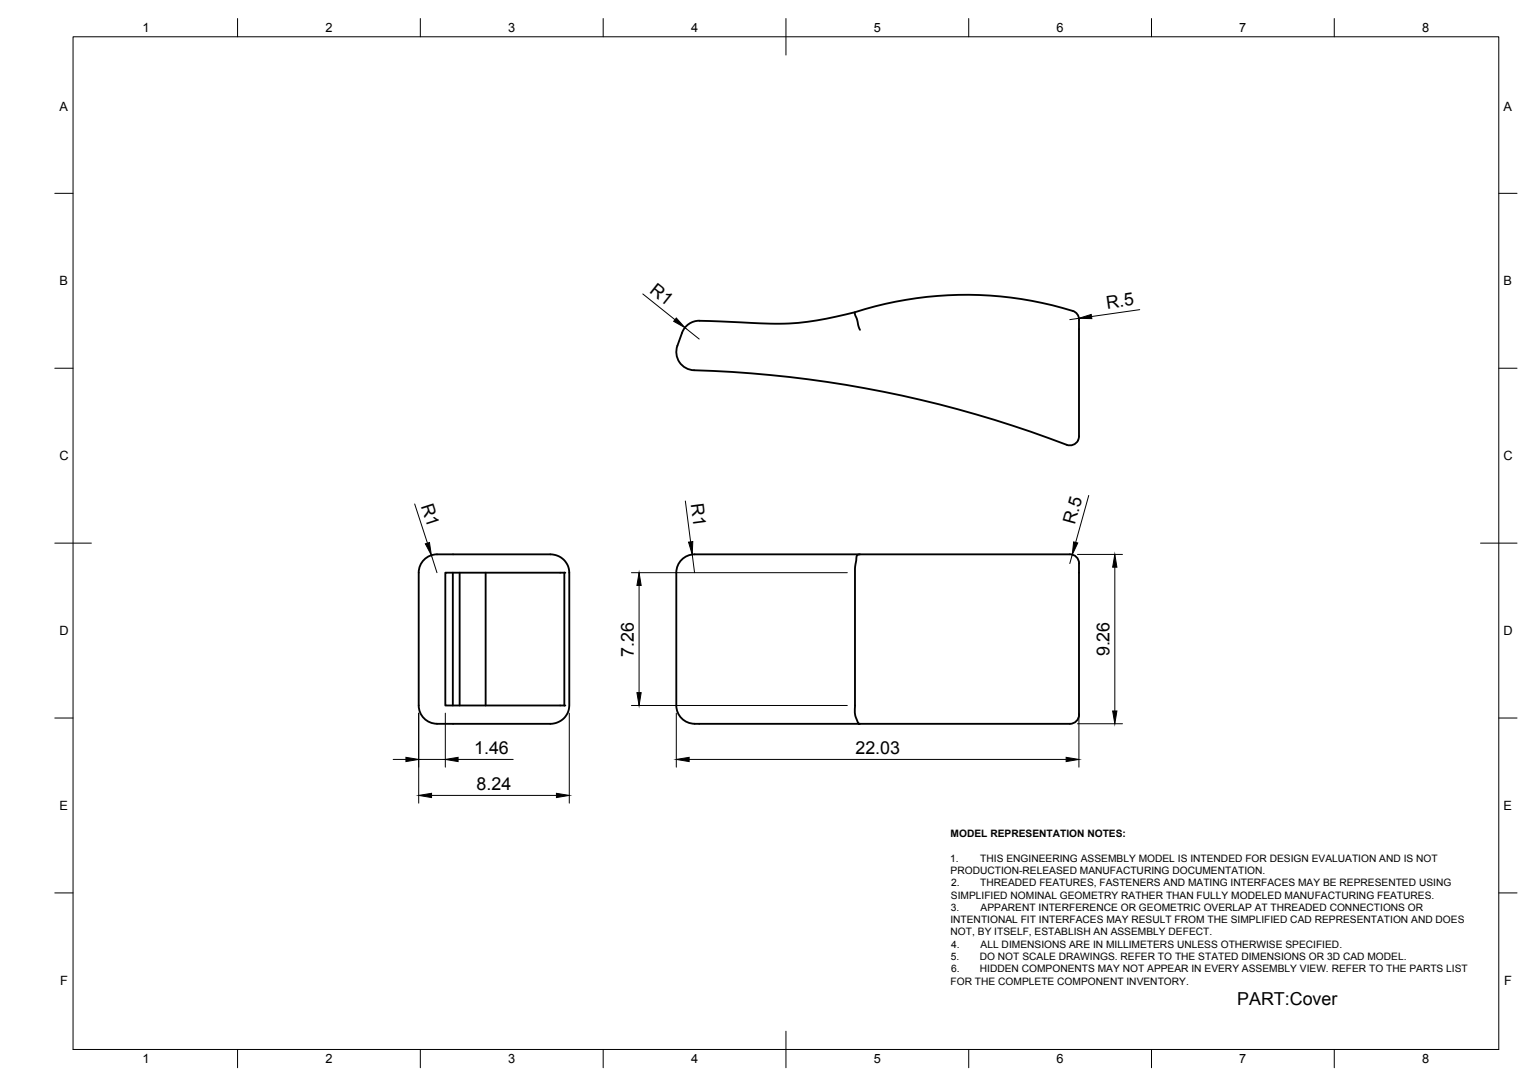
ISO-10303-21;
HEADER;
/* Generated by software containing ST-Developer
 * from STEP Tools, Inc. (www.steptools.com) 
 */

FILE_DESCRIPTION(
/* description */ (''),
/* implementation_level */ '2;1');

FILE_NAME(
/* name */ 'Cover.step',
/* time_stamp */ '2026-10-05T16:20:14-07:00',
/* author */ (''),
/* organization */ (''),
/* preprocessor_version */ 'ST-DEVELOPER v20.2',
/* originating_system */ 'Autodesk Translation Framework v15.15.0.0',
/* authorisation */ '');

FILE_SCHEMA (('AUTOMOTIVE_DESIGN { 1 0 10303 214 3 1 1 }'));
ENDSEC;

DATA;
#10=MECHANICAL_DESIGN_GEOMETRIC_PRESENTATION_REPRESENTATION('',(#255),#23577);
#47=SPHERICAL_SURFACE('',#4635,1.);
#48=SPHERICAL_SURFACE('',#4644,1.);
#49=SPHERICAL_SURFACE('',#4650,1.);
#50=SPHERICAL_SURFACE('',#4654,1.);
#62=B_SPLINE_SURFACE_WITH_KNOTS('',3,3,((#22693,#22694,#22695,#22696,#22697,
#22698),(#22699,#22700,#22701,#22702,#22703,#22704),(#22705,#22706,#22707,
#22708,#22709,#22710),(#22711,#22712,#22713,#22714,#22715,#22716),(#22717,
#22718,#22719,#22720,#22721,#22722),(#22723,#22724,#22725,#22726,#22727,
#22728)),.UNSPECIFIED.,.F.,.F.,.F.,(4,1,1,4),(4,1,1,4),(0.,0.285714285714286,
0.571428571428571,1.00003411570466),(-3.41157046611592E-5,0.0348511435350236,
0.0580852392250393,0.0813534506197162),.UNSPECIFIED.);
#63=B_SPLINE_SURFACE_WITH_KNOTS('',3,3,((#22783,#22784,#22785,#22786,#22787,
#22788),(#22789,#22790,#22791,#22792,#22793,#22794),(#22795,#22796,#22797,
#22798,#22799,#22800),(#22801,#22802,#22803,#22804,#22805,#22806),(#22807,
#22808,#22809,#22810,#22811,#22812),(#22813,#22814,#22815,#22816,#22817,
#22818)),.UNSPECIFIED.,.F.,.F.,.F.,(4,1,1,4),(4,1,1,4),(0.,0.285714285714286,
0.571428571428571,1.00010679363949),(-0.000106793639489728,0.0232340956900158,
0.0348511435350236,0.0814261285545448),.UNSPECIFIED.);
#64=B_SPLINE_SURFACE_WITH_KNOTS('',3,3,((#22879,#22880,#22881,#22882,#22883,
#22884),(#22885,#22886,#22887,#22888,#22889,#22890),(#22891,#22892,#22893,
#22894,#22895,#22896),(#22897,#22898,#22899,#22900,#22901,#22902),(#22903,
#22904,#22905,#22906,#22907,#22908)),.UNSPECIFIED.,.F.,.F.,.F.,(4,1,4),
(4,1,1,4),(0.,0.5,1.),(0.,0.0344711845244392,0.0574519742073987,0.0804327638903581),
 .UNSPECIFIED.);
#65=B_SPLINE_SURFACE_WITH_KNOTS('',3,3,((#22930,#22931,#22932,#22933,#22934),
(#22935,#22936,#22937,#22938,#22939),(#22940,#22941,#22942,#22943,#22944),
(#22945,#22946,#22947,#22948,#22949),(#22950,#22951,#22952,#22953,#22954)),
 .UNSPECIFIED.,.F.,.F.,.F.,(4,1,4),(4,1,4),(0.,0.5,1.),(0.,0.0344716480101997,
0.0804338453571326),.UNSPECIFIED.);
#66=B_SPLINE_SURFACE_WITH_KNOTS('',3,3,((#23009,#23010,#23011,#23012,#23013,
#23014,#23015,#23016,#23017,#23018,#23019),(#23020,#23021,#23022,#23023,
#23024,#23025,#23026,#23027,#23028,#23029,#23030),(#23031,#23032,#23033,
#23034,#23035,#23036,#23037,#23038,#23039,#23040,#23041),(#23042,#23043,
#23044,#23045,#23046,#23047,#23048,#23049,#23050,#23051,#23052),(#23053,
#23054,#23055,#23056,#23057,#23058,#23059,#23060,#23061,#23062,#23063)),
 .UNSPECIFIED.,.F.,.F.,.F.,(4,1,4),(4,2,1,1,1,1,1,4),(0.,0.571428571428571,
1.),(-0.00337447822144074,0.,0.252271193732039,0.378406790598058,0.504542387464077,
0.630677984330096,0.756813581196116,0.882949178062135),.UNSPECIFIED.);
#67=B_SPLINE_SURFACE_WITH_KNOTS('',3,1,((#23117,#23118),(#23119,#23120),
(#23121,#23122),(#23123,#23124),(#23125,#23126)),.UNSPECIFIED.,.F.,.F.,
 .F.,(4,1,4),(2,2),(0.,0.5,1.),(0.,0.8715982725842),.UNSPECIFIED.);
#68=B_SPLINE_SURFACE_WITH_KNOTS('',5,1,((#23132,#23133),(#23134,#23135),
(#23136,#23137),(#23138,#23139),(#23140,#23141),(#23142,#23143),(#23144,
#23145),(#23146,#23147),(#23148,#23149),(#23150,#23151),(#23152,#23153),
(#23154,#23155),(#23156,#23157),(#23158,#23159),(#23160,#23161),(#23162,
#23163),(#23164,#23165),(#23166,#23167),(#23168,#23169),(#23170,#23171)),
 .UNSPECIFIED.,.F.,.F.,.F.,(6,1,1,1,1,1,1,1,1,1,1,1,1,1,1,6),(2,2),(0.,
0.0666666666666667,0.133333333333333,0.2,0.266666666666667,0.333333333333333,
0.4,0.466666666666667,0.533333333333333,0.6,0.666666666666667,0.733333333333333,
0.8,0.866666666666667,0.933333333333333,1.),(0.,1.1115982725842),
 .UNSPECIFIED.);
#69=B_SPLINE_SURFACE_WITH_KNOTS('',3,3,((#23214,#23215,#23216,#23217,#23218,
#23219,#23220,#23221,#23222,#23223),(#23224,#23225,#23226,#23227,#23228,
#23229,#23230,#23231,#23232,#23233),(#23234,#23235,#23236,#23237,#23238,
#23239,#23240,#23241,#23242,#23243),(#23244,#23245,#23246,#23247,#23248,
#23249,#23250,#23251,#23252,#23253),(#23254,#23255,#23256,#23257,#23258,
#23259,#23260,#23261,#23262,#23263)),.UNSPECIFIED.,.F.,.F.,.F.,(4,1,4),
(4,2,1,1,1,1,4),(0.,0.571428571428571,1.),(-0.00337447822145283,0.,0.176589835612662,
0.353179671225324,0.529769506837986,0.706359342450648,0.88294917806331),
 .UNSPECIFIED.);
#70=B_SPLINE_SURFACE_WITH_KNOTS('',5,1,((#23446,#23447),(#23448,#23449),
(#23450,#23451),(#23452,#23453),(#23454,#23455),(#23456,#23457),(#23458,
#23459),(#23460,#23461),(#23462,#23463),(#23464,#23465),(#23466,#23467),
(#23468,#23469),(#23470,#23471),(#23472,#23473),(#23474,#23475),(#23476,
#23477),(#23478,#23479),(#23480,#23481),(#23482,#23483),(#23484,#23485),
(#23486,#23487),(#23488,#23489),(#23490,#23491),(#23492,#23493),(#23494,
#23495),(#23496,#23497),(#23498,#23499),(#23500,#23501),(#23502,#23503),
(#23504,#23505),(#23506,#23507),(#23508,#23509),(#23510,#23511)),
 .UNSPECIFIED.,.F.,.F.,.F.,(6,1,1,1,1,1,1,1,1,1,1,1,1,1,1,1,1,1,1,1,1,1,
1,1,1,1,1,1,6),(2,2),(0.45747490134806,0.46,0.48,0.5,0.52,0.54,0.56,0.58,
0.6,0.62,0.64,0.66,0.68,0.7,0.72,0.74,0.76,0.78,0.8,0.82,0.84,0.86,0.88,
0.9,0.92,0.940000000000001,0.960000000000001,0.980000000000001,0.998665134312148),
(0.,0.931560000000001),.UNSPECIFIED.);
#191=B_SPLINE_CURVE_WITH_KNOTS('',3,(#22733,#22734,#22735,#22736,#22737,
#22738,#22739,#22740,#22741,#22742,#22743,#22744,#22745,#22746,#22747,#22748,
#22749,#22750,#22751,#22752,#22753,#22754,#22755,#22756,#22757,#22758,#22759,
#22760,#22761,#22762,#22763,#22764,#22765,#22766,#22767,#22768,#22769,#22770,
#22771,#22772),.UNSPECIFIED.,.F.,.F.,(4,3,3,3,3,3,3,3,3,3,3,3,3,4),(-0.081319334915055,
-0.0753389837263114,-0.0693564459716813,-0.0633597360066557,-0.0580852392250393,
-0.0515874996582905,-0.0450649979609627,-0.0384986686708182,-0.0348511435350236,
-0.0271955520394085,-0.0193080379818354,-0.0113079400461875,-0.00319973662204704,
0.),.UNSPECIFIED.);
#192=B_SPLINE_CURVE_WITH_KNOTS('',3,(#22776,#22777,#22778,#22779,#22780,
#22781),.UNSPECIFIED.,.F.,.F.,(4,1,1,4),(0.,0.0348511435350236,0.0580852392250393,
0.081319334915055),.UNSPECIFIED.);
#193=B_SPLINE_CURVE_WITH_KNOTS('',3,(#22823,#22824,#22825,#22826,#22827,
#22828,#22829,#22830,#22831,#22832,#22833,#22834,#22835,#22836,#22837,#22838,
#22839,#22840,#22841,#22842,#22843,#22844,#22845,#22846,#22847,#22848,#22849,
#22850,#22851,#22852,#22853,#22854,#22855,#22856,#22857,#22858,#22859,#22860,
#22861,#22862),.UNSPECIFIED.,.F.,.F.,(4,3,3,3,3,3,3,3,3,3,3,3,3,4),(-0.0813193349150551,
-0.0734858773515304,-0.0657143436353313,-0.0579985436102544,-0.0504671957638769,
-0.0426591696494502,-0.0353839636779,-0.0348511435350236,-0.0290426196125197,
-0.0232340956900158,-0.016758297070707,-0.010297938217042,-0.00385507197155476,
0.),.UNSPECIFIED.);
#194=B_SPLINE_CURVE_WITH_KNOTS('',3,(#22867,#22868,#22869,#22870,#22871,
#22872),.UNSPECIFIED.,.F.,.F.,(4,1,1,4),(0.,0.0232340956900158,0.0348511435350236,
0.0813193349150551),.UNSPECIFIED.);
#195=B_SPLINE_CURVE_WITH_KNOTS('',3,(#22912,#22913,#22914,#22915,#22916,
#22917),.UNSPECIFIED.,.F.,.F.,(4,1,1,4),(-0.0804327638903581,-0.0574519742073987,
-0.0344711845244392,0.),.UNSPECIFIED.);
#196=B_SPLINE_CURVE_WITH_KNOTS('',3,(#22918,#22919,#22920,#22921,#22922,
#22923),.UNSPECIFIED.,.F.,.F.,(4,1,1,4),(0.,0.0344711845244392,0.0574519742073987,
0.0804327638903581),.UNSPECIFIED.);
#197=B_SPLINE_CURVE_WITH_KNOTS('',3,(#22958,#22959,#22960,#22961,#22962),
 .UNSPECIFIED.,.F.,.F.,(4,1,4),(-0.0804338453571326,-0.0344716480101997,
0.),.UNSPECIFIED.);
#198=B_SPLINE_CURVE_WITH_KNOTS('',3,(#22963,#22964,#22965,#22966,#22967),
 .UNSPECIFIED.,.F.,.F.,(4,1,4),(0.,0.0344716480101997,0.0804338453571326),
 .UNSPECIFIED.);
#199=B_SPLINE_CURVE_WITH_KNOTS('',3,(#22980,#22981,#22982,#22983,#22984,
#22985,#22986,#22987,#22988,#22989),.UNSPECIFIED.,.F.,.F.,(4,2,1,1,1,1,
4),(-0.00337447822145283,0.,0.176589835612662,0.353179671225324,0.529769506837986,
0.706359342450648,0.88294917806331),.UNSPECIFIED.);
#200=B_SPLINE_CURVE_WITH_KNOTS('',3,(#23066,#23067,#23068,#23069,#23070,
#23071,#23072,#23073,#23074),.UNSPECIFIED.,.F.,.F.,(4,1,1,1,1,1,4),(2.79137390763681E-5,
0.252271193732039,0.378406790598058,0.504542387464077,0.630677984330096,
0.756813581196116,0.882949178062135),.UNSPECIFIED.);
#201=B_SPLINE_CURVE_WITH_KNOTS('',3,(#23078,#23079,#23080,#23081,#23082,
#23083,#23084,#23085,#23086,#23087,#23088),.UNSPECIFIED.,.F.,.F.,(4,1,1,
1,1,1,2,4),(-0.882949178062135,-0.756813581196116,-0.630677984330096,-0.504542387464077,
-0.378406790598058,-0.252271193732039,0.,0.00337447822144074),
 .UNSPECIFIED.);
#202=B_SPLINE_CURVE_WITH_KNOTS('',3,(#23089,#23090,#23091,#23092,#23093,
#23094,#23095,#23096,#23097,#23098,#23099,#23100,#23101,#23102,#23103,#23104),
 .UNSPECIFIED.,.F.,.F.,(4,2,2,2,2,2,2,4),(-0.000760845488671771,0.,0.0228705421389603,
0.0452951187281299,0.0845262515009002,0.116879048291215,0.130924332719927,
0.145498548542211),.UNSPECIFIED.);
#203=B_SPLINE_CURVE_WITH_KNOTS('',5,(#23174,#23175,#23176,#23177,#23178,
#23179,#23180,#23181,#23182,#23183,#23184,#23185,#23186,#23187,#23188,#23189,
#23190,#23191,#23192),.UNSPECIFIED.,.F.,.F.,(6,1,1,1,1,1,1,1,1,1,1,1,1,
1,6),(-0.931895129353616,-0.866666666666667,-0.8,-0.733333333333333,-0.666666666666667,
-0.6,-0.533333333333333,-0.466666666666667,-0.4,-0.333333333333333,-0.266666666666667,
-0.2,-0.133333333333333,-0.0666666666666667,-3.17880566490557E-7),
 .UNSPECIFIED.);
#204=B_SPLINE_CURVE_WITH_KNOTS('',3,(#23197,#23198,#23199,#23200,#23201,
#23202,#23203,#23204,#23205,#23206,#23207,#23208,#23209,#23210,#23211,#23212),
 .UNSPECIFIED.,.F.,.F.,(4,2,2,2,2,2,2,4),(-0.0825251055196344,-0.08233525228657,
-0.075900251435362,-0.0686308963896873,-0.0574260404457226,-0.0407017513607544,
-0.0210184504217403,0.),.UNSPECIFIED.);
#205=B_SPLINE_CURVE_WITH_KNOTS('',3,(#23278,#23279,#23280,#23281,#23282,
#23283,#23284,#23285,#23286,#23287,#23288,#23289,#23290,#23291,#23292,#23293,
#23294,#23295,#23296,#23297,#23298,#23299,#23300,#23301,#23302,#23303,#23304,
#23305,#23306,#23307,#23308,#23309,#23310,#23311,#23312,#23313,#23314,#23315,
#23316,#23317,#23318,#23319,#23320,#23321,#23322,#23323,#23324,#23325,#23326,
#23327,#23328,#23329,#23330,#23331,#23332,#23333,#23334,#23335,#23336,#23337,
#23338,#23339,#23340,#23341,#23342,#23343,#23344,#23345,#23346,#23347,#23348,
#23349,#23350,#23351,#23352,#23353,#23354,#23355,#23356,#23357,#23358,#23359,
#23360,#23361,#23362,#23363,#23364,#23365,#23366,#23367,#23368,#23369,#23370,
#23371,#23372,#23373,#23374,#23375,#23376,#23377,#23378,#23379,#23380,#23381,
#23382,#23383,#23384,#23385,#23386,#23387,#23388,#23389,#23390,#23391,#23392,
#23393,#23394,#23395,#23396,#23397,#23398,#23399,#23400,#23401,#23402,#23403,
#23404,#23405,#23406,#23407,#23408,#23409,#23410,#23411,#23412,#23413,#23414,
#23415,#23416,#23417,#23418,#23419,#23420,#23421,#23422,#23423,#23424,#23425,
#23426,#23427,#23428,#23429,#23430,#23431,#23432,#23433,#23434),
 .UNSPECIFIED.,.F.,.F.,(4,3,3,3,3,3,3,3,3,3,3,3,3,3,3,3,3,3,3,3,3,3,3,3,
3,3,3,3,3,3,3,3,3,3,3,3,3,3,3,3,3,3,3,3,3,3,3,3,3,3,3,3,4),(-4.43919555064984,
-4.31351752310522,-4.21748497989632,-4.13039569871212,-4.04917309818115,
-3.97216182461211,-3.89780976908328,-3.82536061976307,-3.75520238328067,
-3.68765512117113,-3.62163278915582,-3.55440616562861,-3.48496721361178,
-3.40927574040849,-3.3121488002462,-3.22434990344501,-3.15109446525443,
-3.08492269429087,-3.02341966724156,-2.96461369321188,-2.90551252744871,
-2.84539597265316,-2.78402646194644,-2.72077433031378,-2.65518089902205,
-2.58678643782235,-2.51494173113323,-2.4351726591892,-2.3469342569877,-2.24741963324518,
-2.1576576071755,-2.0742009601071,-1.99319641369387,-1.91148636863784,-1.82737832465568,
-1.74166088715984,-1.65491799562197,-1.56650259700221,-1.4759044479693,
-1.3822422658407,-1.28644440225838,-1.18824460058421,-1.087792421038,-0.985316046032208,
-0.877949096049762,-0.75542711973491,-0.615520892462394,-0.46127383549543,
-0.336504337401264,-0.222259848570182,-0.111129924285091,-0.0120794939036124,
0.),.UNSPECIFIED.);
#206=B_SPLINE_CURVE_WITH_KNOTS('',5,(#23512,#23513,#23514,#23515,#23516,
#23517,#23518,#23519,#23520,#23521,#23522,#23523,#23524,#23525,#23526,#23527,
#23528,#23529,#23530,#23531,#23532,#23533,#23534,#23535,#23536,#23537,#23538,
#23539,#23540,#23541,#23542,#23543,#23544),.UNSPECIFIED.,.F.,.F.,(6,1,1,
1,1,1,1,1,1,1,1,1,1,1,1,1,1,1,1,1,1,1,1,1,1,1,1,1,6),(-0.998665134312148,
-0.980000000000001,-0.960000000000001,-0.940000000000001,-0.92,-0.9,-0.88,
-0.86,-0.84,-0.82,-0.8,-0.78,-0.76,-0.74,-0.72,-0.7,-0.68,-0.66,-0.64,-0.62,
-0.6,-0.58,-0.56,-0.54,-0.52,-0.5,-0.48,-0.46,-0.45747490134806),
 .UNSPECIFIED.);
#211=ELLIPSE('',#4610,0.440642274355316,0.384283137019794);
#212=ELLIPSE('',#4613,0.440642274355316,0.384283137019794);
#225=TOROIDAL_SURFACE('',#4625,62.8868723549169,1.);
#226=TOROIDAL_SURFACE('',#4630,62.8868723549169,1.);
#227=TOROIDAL_SURFACE('',#4638,18.7866355153418,1.);
#228=TOROIDAL_SURFACE('',#4647,18.7866355153418,1.);
#237=SHAPE_REPRESENTATION_RELATIONSHIP('SRR','None',#23620,#246);
#246=ADVANCED_BREP_SHAPE_REPRESENTATION('',(#264),#23576);
#255=STYLED_ITEM('',(#23669),#264);
#264=MANIFOLD_SOLID_BREP('Body1',#4165);
#389=PLANE('',#4622);
#390=PLANE('',#4633);
#391=PLANE('',#4646);
#392=PLANE('',#4657);
#393=PLANE('',#4658);
#394=PLANE('',#4662);
#395=PLANE('',#4663);
#588=FACE_OUTER_BOUND('',#849,.T.);
#589=FACE_OUTER_BOUND('',#850,.T.);
#590=FACE_OUTER_BOUND('',#851,.T.);
#591=FACE_OUTER_BOUND('',#852,.T.);
#592=FACE_OUTER_BOUND('',#853,.T.);
#593=FACE_OUTER_BOUND('',#854,.T.);
#594=FACE_OUTER_BOUND('',#855,.T.);
#595=FACE_OUTER_BOUND('',#856,.T.);
#596=FACE_OUTER_BOUND('',#857,.T.);
#597=FACE_OUTER_BOUND('',#858,.T.);
#598=FACE_OUTER_BOUND('',#859,.T.);
#599=FACE_OUTER_BOUND('',#860,.T.);
#600=FACE_OUTER_BOUND('',#861,.T.);
#601=FACE_OUTER_BOUND('',#862,.T.);
#602=FACE_OUTER_BOUND('',#863,.T.);
#603=FACE_OUTER_BOUND('',#864,.T.);
#604=FACE_OUTER_BOUND('',#865,.T.);
#605=FACE_OUTER_BOUND('',#866,.T.);
#606=FACE_OUTER_BOUND('',#867,.T.);
#607=FACE_OUTER_BOUND('',#868,.T.);
#608=FACE_OUTER_BOUND('',#869,.T.);
#609=FACE_OUTER_BOUND('',#870,.T.);
#610=FACE_OUTER_BOUND('',#871,.T.);
#611=FACE_OUTER_BOUND('',#872,.T.);
#612=FACE_OUTER_BOUND('',#873,.T.);
#613=FACE_OUTER_BOUND('',#874,.T.);
#614=FACE_OUTER_BOUND('',#875,.T.);
#615=FACE_OUTER_BOUND('',#876,.T.);
#616=FACE_OUTER_BOUND('',#877,.T.);
#617=FACE_OUTER_BOUND('',#878,.T.);
#618=FACE_OUTER_BOUND('',#879,.T.);
#619=FACE_OUTER_BOUND('',#880,.T.);
#620=FACE_OUTER_BOUND('',#881,.T.);
#621=FACE_OUTER_BOUND('',#882,.T.);
#849=EDGE_LOOP('',(#3697,#3698,#3699,#3700,#3701));
#850=EDGE_LOOP('',(#3702,#3703,#3704,#3705,#3706));
#851=EDGE_LOOP('',(#3707,#3708,#3709,#3710));
#852=EDGE_LOOP('',(#3711,#3712,#3713,#3714));
#853=EDGE_LOOP('',(#3715,#3716,#3717,#3718));
#854=EDGE_LOOP('',(#3719,#3720,#3721,#3722));
#855=EDGE_LOOP('',(#3723,#3724,#3725,#3726));
#856=EDGE_LOOP('',(#3727,#3728,#3729,#3730));
#857=EDGE_LOOP('',(#3731,#3732,#3733,#3734,#3735));
#858=EDGE_LOOP('',(#3736,#3737,#3738,#3739));
#859=EDGE_LOOP('',(#3740,#3741,#3742,#3743));
#860=EDGE_LOOP('',(#3744,#3745,#3746,#3747));
#861=EDGE_LOOP('',(#3748,#3749,#3750,#3751,#3752,#3753,#3754,#3755,#3756,
#3757));
#862=EDGE_LOOP('',(#3758,#3759,#3760,#3761));
#863=EDGE_LOOP('',(#3762,#3763,#3764));
#864=EDGE_LOOP('',(#3765,#3766,#3767,#3768));
#865=EDGE_LOOP('',(#3769,#3770,#3771,#3772));
#866=EDGE_LOOP('',(#3773,#3774,#3775,#3776));
#867=EDGE_LOOP('',(#3777,#3778,#3779,#3780));
#868=EDGE_LOOP('',(#3781,#3782,#3783));
#869=EDGE_LOOP('',(#3784,#3785,#3786,#3787,#3788));
#870=EDGE_LOOP('',(#3789,#3790,#3791,#3792));
#871=EDGE_LOOP('',(#3793,#3794,#3795,#3796));
#872=EDGE_LOOP('',(#3797,#3798,#3799));
#873=EDGE_LOOP('',(#3800,#3801,#3802,#3803));
#874=EDGE_LOOP('',(#3804,#3805,#3806));
#875=EDGE_LOOP('',(#3807,#3808,#3809,#3810));
#876=EDGE_LOOP('',(#3811,#3812,#3813,#3814));
#877=EDGE_LOOP('',(#3815,#3816,#3817,#3818,#3819));
#878=EDGE_LOOP('',(#3820,#3821,#3822,#3823));
#879=EDGE_LOOP('',(#3824,#3825,#3826,#3827));
#880=EDGE_LOOP('',(#3828,#3829,#3830,#3831));
#881=EDGE_LOOP('',(#3832,#3833,#3834,#3835,#3836));
#882=EDGE_LOOP('',(#3837,#3838,#3839,#3840));
#1144=LINE('',#22877,#1429);
#1145=LINE('',#22878,#1430);
#1146=LINE('',#22928,#1431);
#1147=LINE('',#22929,#1432);
#1148=LINE('',#22969,#1433);
#1149=LINE('',#22970,#1434);
#1150=LINE('',#22972,#1435);
#1151=LINE('',#22973,#1436);
#1152=LINE('',#22978,#1437);
#1153=LINE('',#22998,#1438);
#1154=LINE('',#23005,#1439);
#1155=LINE('',#23007,#1440);
#1156=LINE('',#23008,#1441);
#1157=LINE('',#23114,#1442);
#1158=LINE('',#23116,#1443);
#1159=LINE('',#23128,#1444);
#1160=LINE('',#23131,#1445);
#1161=LINE('',#23173,#1446);
#1162=LINE('',#23270,#1447);
#1163=LINE('',#23274,#1448);
#1164=LINE('',#23436,#1449);
#1165=LINE('',#23440,#1450);
#1166=LINE('',#23444,#1451);
#1167=LINE('',#23445,#1452);
#1429=VECTOR('',#5635,10.);
#1430=VECTOR('',#5636,10.);
#1431=VECTOR('',#5643,10.);
#1432=VECTOR('',#5644,10.);
#1433=VECTOR('',#5649,10.);
#1434=VECTOR('',#5650,10.);
#1435=VECTOR('',#5653,10.);
#1436=VECTOR('',#5654,10.);
#1437=VECTOR('',#5659,10.);
#1438=VECTOR('',#5672,10.);
#1439=VECTOR('',#5681,10.);
#1440=VECTOR('',#5682,10.);
#1441=VECTOR('',#5683,10.);
#1442=VECTOR('',#5700,10.);
#1443=VECTOR('',#5703,10.);
#1444=VECTOR('',#5704,10.);
#1445=VECTOR('',#5707,10.);
#1446=VECTOR('',#5708,10.);
#1447=VECTOR('',#5729,10.);
#1448=VECTOR('',#5736,10.);
#1449=VECTOR('',#5741,10.);
#1450=VECTOR('',#5746,10.);
#1451=VECTOR('',#5751,10.);
#1452=VECTOR('',#5752,10.);
#1598=CIRCLE('',#4608,0.499999999999996);
#1599=CIRCLE('',#4609,0.5);
#1600=CIRCLE('',#4611,0.499999999999996);
#1601=CIRCLE('',#4612,0.499999999999992);
#1602=CIRCLE('',#4615,0.499999999999995);
#1603=CIRCLE('',#4616,0.499999999999996);
#1604=CIRCLE('',#4618,0.499999999999987);
#1605=CIRCLE('',#4619,0.499999999999996);
#1606=CIRCLE('',#4623,62.8868723549169);
#1607=CIRCLE('',#4624,18.7866355153418);
#1608=CIRCLE('',#4626,61.8868723549169);
#1609=CIRCLE('',#4627,0.999999999999999);
#1610=CIRCLE('',#4629,61.8868723549169);
#1611=CIRCLE('',#4631,62.8868723549169);
#1612=CIRCLE('',#4632,1.);
#1613=CIRCLE('',#4634,1.);
#1614=CIRCLE('',#4636,1.00000000000001);
#1615=CIRCLE('',#4637,1.);
#1616=CIRCLE('',#4639,19.7866355153418);
#1617=CIRCLE('',#4640,18.7866355153418);
#1618=CIRCLE('',#4642,1.);
#1619=CIRCLE('',#4643,1.00000000000001);
#1620=CIRCLE('',#4645,0.999999999999998);
#1621=CIRCLE('',#4648,19.7866355153418);
#1622=CIRCLE('',#4649,1.);
#1623=CIRCLE('',#4651,1.);
#1624=CIRCLE('',#4653,1.);
#1625=CIRCLE('',#4655,0.999999999999998);
#1626=CIRCLE('',#4659,62.3332952479768);
#1627=CIRCLE('',#4661,62.3332952479768);
#1995=VERTEX_POINT('',#22729);
#1996=VERTEX_POINT('',#22730);
#1997=VERTEX_POINT('',#22732);
#1998=VERTEX_POINT('',#22773);
#1999=VERTEX_POINT('',#22775);
#2000=VERTEX_POINT('',#22819);
#2001=VERTEX_POINT('',#22820);
#2002=VERTEX_POINT('',#22822);
#2003=VERTEX_POINT('',#22863);
#2004=VERTEX_POINT('',#22865);
#2005=VERTEX_POINT('',#22874);
#2006=VERTEX_POINT('',#22875);
#2007=VERTEX_POINT('',#22909);
#2008=VERTEX_POINT('',#22910);
#2009=VERTEX_POINT('',#22925);
#2010=VERTEX_POINT('',#22926);
#2011=VERTEX_POINT('',#22955);
#2012=VERTEX_POINT('',#22956);
#2013=VERTEX_POINT('',#22975);
#2014=VERTEX_POINT('',#22977);
#2015=VERTEX_POINT('',#22979);
#2016=VERTEX_POINT('',#22992);
#2017=VERTEX_POINT('',#22996);
#2018=VERTEX_POINT('',#23000);
#2019=VERTEX_POINT('',#23004);
#2020=VERTEX_POINT('',#23006);
#2021=VERTEX_POINT('',#23064);
#2022=VERTEX_POINT('',#23065);
#2023=VERTEX_POINT('',#23075);
#2024=VERTEX_POINT('',#23077);
#2025=VERTEX_POINT('',#23106);
#2026=VERTEX_POINT('',#23113);
#2027=VERTEX_POINT('',#23127);
#2028=VERTEX_POINT('',#23129);
#2029=VERTEX_POINT('',#23172);
#2030=VERTEX_POINT('',#23268);
#2031=VERTEX_POINT('',#23277);
#2032=VERTEX_POINT('',#23435);
#2033=VERTEX_POINT('',#23439);
#2034=VERTEX_POINT('',#23443);
#2565=EDGE_CURVE('',#1995,#1996,#1598,.T.);
#2566=EDGE_CURVE('',#1996,#1997,#191,.T.);
#2567=EDGE_CURVE('',#1997,#1998,#1599,.T.);
#2568=EDGE_CURVE('',#1998,#1999,#192,.T.);
#2569=EDGE_CURVE('',#1999,#1995,#211,.T.);
#2570=EDGE_CURVE('',#2000,#2001,#1600,.T.);
#2571=EDGE_CURVE('',#2001,#2002,#193,.T.);
#2572=EDGE_CURVE('',#2002,#2003,#1601,.T.);
#2573=EDGE_CURVE('',#2003,#2004,#212,.T.);
#2574=EDGE_CURVE('',#2004,#2000,#194,.T.);
#2575=EDGE_CURVE('',#2005,#2006,#1602,.T.);
#2576=EDGE_CURVE('',#2006,#2001,#1144,.T.);
#2577=EDGE_CURVE('',#2000,#2005,#1145,.T.);
#2578=EDGE_CURVE('',#2007,#2008,#1603,.T.);
#2579=EDGE_CURVE('',#2008,#2006,#195,.T.);
#2580=EDGE_CURVE('',#2005,#2007,#196,.T.);
#2581=EDGE_CURVE('',#2009,#2010,#1604,.T.);
#2582=EDGE_CURVE('',#2010,#2008,#1146,.T.);
#2583=EDGE_CURVE('',#2007,#2009,#1147,.T.);
#2584=EDGE_CURVE('',#2011,#2012,#1605,.T.);
#2585=EDGE_CURVE('',#2012,#2010,#197,.T.);
#2586=EDGE_CURVE('',#2009,#2011,#198,.T.);
#2587=EDGE_CURVE('',#2011,#1998,#1148,.T.);
#2588=EDGE_CURVE('',#1997,#2012,#1149,.T.);
#2589=EDGE_CURVE('',#1995,#2003,#1150,.T.);
#2590=EDGE_CURVE('',#2002,#1996,#1151,.T.);
#2591=EDGE_CURVE('',#2013,#1997,#1606,.T.);
#2592=EDGE_CURVE('',#2014,#2013,#1152,.T.);
#2593=EDGE_CURVE('',#2015,#2014,#199,.T.);
#2594=EDGE_CURVE('',#2012,#2015,#1607,.T.);
#2595=EDGE_CURVE('',#1996,#2016,#1608,.T.);
#2596=EDGE_CURVE('',#2016,#2013,#1609,.T.);
#2597=EDGE_CURVE('',#2017,#2002,#1610,.T.);
#2598=EDGE_CURVE('',#2016,#2017,#1153,.T.);
#2599=EDGE_CURVE('',#2001,#2018,#1611,.T.);
#2600=EDGE_CURVE('',#2018,#2017,#1612,.T.);
#2601=EDGE_CURVE('',#2004,#2019,#1154,.T.);
#2602=EDGE_CURVE('',#2019,#2020,#1155,.T.);
#2603=EDGE_CURVE('',#1999,#2020,#1156,.T.);
#2604=EDGE_CURVE('',#2021,#2022,#200,.T.);
#2605=EDGE_CURVE('',#2022,#2023,#1613,.T.);
#2606=EDGE_CURVE('',#2023,#2024,#201,.T.);
#2607=EDGE_CURVE('',#2024,#2021,#202,.T.);
#2608=EDGE_CURVE('',#2022,#2025,#1614,.T.);
#2609=EDGE_CURVE('',#2025,#2023,#1615,.T.);
#2610=EDGE_CURVE('',#2008,#2021,#1616,.T.);
#2611=EDGE_CURVE('',#2024,#2006,#1617,.T.);
#2612=EDGE_CURVE('',#2025,#2026,#1157,.T.);
#2613=EDGE_CURVE('',#2018,#2026,#1618,.T.);
#2614=EDGE_CURVE('',#2018,#2023,#1158,.T.);
#2615=EDGE_CURVE('',#2022,#2027,#1159,.T.);
#2616=EDGE_CURVE('',#2028,#2027,#1619,.T.);
#2617=EDGE_CURVE('',#2028,#2025,#1160,.T.);
#2618=EDGE_CURVE('',#2029,#2021,#1161,.T.);
#2619=EDGE_CURVE('',#2027,#2029,#203,.T.);
#2620=EDGE_CURVE('',#2026,#2017,#1620,.T.);
#2621=EDGE_CURVE('',#2015,#2029,#204,.T.);
#2622=EDGE_CURVE('',#2029,#2010,#1621,.T.);
#2623=EDGE_CURVE('',#2014,#2027,#1622,.T.);
#2624=EDGE_CURVE('',#2014,#2028,#1623,.T.);
#2625=EDGE_CURVE('',#2030,#2013,#1624,.T.);
#2626=EDGE_CURVE('',#2030,#2028,#1162,.T.);
#2627=EDGE_CURVE('',#2016,#2030,#1625,.T.);
#2628=EDGE_CURVE('',#2026,#2030,#1163,.T.);
#2629=EDGE_CURVE('',#2031,#2020,#205,.T.);
#2630=EDGE_CURVE('',#2032,#2031,#1164,.T.);
#2631=EDGE_CURVE('',#1995,#2032,#1626,.T.);
#2632=EDGE_CURVE('',#2033,#2032,#1165,.T.);
#2633=EDGE_CURVE('',#2003,#2033,#1627,.T.);
#2634=EDGE_CURVE('',#2034,#2031,#1166,.T.);
#2635=EDGE_CURVE('',#2033,#2034,#1167,.T.);
#2636=EDGE_CURVE('',#2034,#2019,#206,.T.);
#3697=ORIENTED_EDGE('',*,*,#2565,.T.);
#3698=ORIENTED_EDGE('',*,*,#2566,.T.);
#3699=ORIENTED_EDGE('',*,*,#2567,.T.);
#3700=ORIENTED_EDGE('',*,*,#2568,.T.);
#3701=ORIENTED_EDGE('',*,*,#2569,.T.);
#3702=ORIENTED_EDGE('',*,*,#2570,.T.);
#3703=ORIENTED_EDGE('',*,*,#2571,.T.);
#3704=ORIENTED_EDGE('',*,*,#2572,.T.);
#3705=ORIENTED_EDGE('',*,*,#2573,.T.);
#3706=ORIENTED_EDGE('',*,*,#2574,.T.);
#3707=ORIENTED_EDGE('',*,*,#2575,.T.);
#3708=ORIENTED_EDGE('',*,*,#2576,.T.);
#3709=ORIENTED_EDGE('',*,*,#2570,.F.);
#3710=ORIENTED_EDGE('',*,*,#2577,.T.);
#3711=ORIENTED_EDGE('',*,*,#2578,.T.);
#3712=ORIENTED_EDGE('',*,*,#2579,.T.);
#3713=ORIENTED_EDGE('',*,*,#2575,.F.);
#3714=ORIENTED_EDGE('',*,*,#2580,.T.);
#3715=ORIENTED_EDGE('',*,*,#2581,.T.);
#3716=ORIENTED_EDGE('',*,*,#2582,.T.);
#3717=ORIENTED_EDGE('',*,*,#2578,.F.);
#3718=ORIENTED_EDGE('',*,*,#2583,.T.);
#3719=ORIENTED_EDGE('',*,*,#2584,.T.);
#3720=ORIENTED_EDGE('',*,*,#2585,.T.);
#3721=ORIENTED_EDGE('',*,*,#2581,.F.);
#3722=ORIENTED_EDGE('',*,*,#2586,.T.);
#3723=ORIENTED_EDGE('',*,*,#2584,.F.);
#3724=ORIENTED_EDGE('',*,*,#2587,.T.);
#3725=ORIENTED_EDGE('',*,*,#2567,.F.);
#3726=ORIENTED_EDGE('',*,*,#2588,.T.);
#3727=ORIENTED_EDGE('',*,*,#2589,.T.);
#3728=ORIENTED_EDGE('',*,*,#2572,.F.);
#3729=ORIENTED_EDGE('',*,*,#2590,.T.);
#3730=ORIENTED_EDGE('',*,*,#2565,.F.);
#3731=ORIENTED_EDGE('',*,*,#2588,.F.);
#3732=ORIENTED_EDGE('',*,*,#2591,.F.);
#3733=ORIENTED_EDGE('',*,*,#2592,.F.);
#3734=ORIENTED_EDGE('',*,*,#2593,.F.);
#3735=ORIENTED_EDGE('',*,*,#2594,.F.);
#3736=ORIENTED_EDGE('',*,*,#2566,.F.);
#3737=ORIENTED_EDGE('',*,*,#2595,.T.);
#3738=ORIENTED_EDGE('',*,*,#2596,.T.);
#3739=ORIENTED_EDGE('',*,*,#2591,.T.);
#3740=ORIENTED_EDGE('',*,*,#2590,.F.);
#3741=ORIENTED_EDGE('',*,*,#2597,.F.);
#3742=ORIENTED_EDGE('',*,*,#2598,.F.);
#3743=ORIENTED_EDGE('',*,*,#2595,.F.);
#3744=ORIENTED_EDGE('',*,*,#2571,.F.);
#3745=ORIENTED_EDGE('',*,*,#2599,.T.);
#3746=ORIENTED_EDGE('',*,*,#2600,.T.);
#3747=ORIENTED_EDGE('',*,*,#2597,.T.);
#3748=ORIENTED_EDGE('',*,*,#2568,.F.);
#3749=ORIENTED_EDGE('',*,*,#2587,.F.);
#3750=ORIENTED_EDGE('',*,*,#2586,.F.);
#3751=ORIENTED_EDGE('',*,*,#2583,.F.);
#3752=ORIENTED_EDGE('',*,*,#2580,.F.);
#3753=ORIENTED_EDGE('',*,*,#2577,.F.);
#3754=ORIENTED_EDGE('',*,*,#2574,.F.);
#3755=ORIENTED_EDGE('',*,*,#2601,.T.);
#3756=ORIENTED_EDGE('',*,*,#2602,.T.);
#3757=ORIENTED_EDGE('',*,*,#2603,.F.);
#3758=ORIENTED_EDGE('',*,*,#2604,.T.);
#3759=ORIENTED_EDGE('',*,*,#2605,.T.);
#3760=ORIENTED_EDGE('',*,*,#2606,.T.);
#3761=ORIENTED_EDGE('',*,*,#2607,.T.);
#3762=ORIENTED_EDGE('',*,*,#2605,.F.);
#3763=ORIENTED_EDGE('',*,*,#2608,.T.);
#3764=ORIENTED_EDGE('',*,*,#2609,.T.);
#3765=ORIENTED_EDGE('',*,*,#2579,.F.);
#3766=ORIENTED_EDGE('',*,*,#2610,.T.);
#3767=ORIENTED_EDGE('',*,*,#2607,.F.);
#3768=ORIENTED_EDGE('',*,*,#2611,.T.);
#3769=ORIENTED_EDGE('',*,*,#2609,.F.);
#3770=ORIENTED_EDGE('',*,*,#2612,.T.);
#3771=ORIENTED_EDGE('',*,*,#2613,.F.);
#3772=ORIENTED_EDGE('',*,*,#2614,.T.);
#3773=ORIENTED_EDGE('',*,*,#2608,.F.);
#3774=ORIENTED_EDGE('',*,*,#2615,.T.);
#3775=ORIENTED_EDGE('',*,*,#2616,.F.);
#3776=ORIENTED_EDGE('',*,*,#2617,.T.);
#3777=ORIENTED_EDGE('',*,*,#2604,.F.);
#3778=ORIENTED_EDGE('',*,*,#2618,.F.);
#3779=ORIENTED_EDGE('',*,*,#2619,.F.);
#3780=ORIENTED_EDGE('',*,*,#2615,.F.);
#3781=ORIENTED_EDGE('',*,*,#2600,.F.);
#3782=ORIENTED_EDGE('',*,*,#2613,.T.);
#3783=ORIENTED_EDGE('',*,*,#2620,.T.);
#3784=ORIENTED_EDGE('',*,*,#2576,.F.);
#3785=ORIENTED_EDGE('',*,*,#2611,.F.);
#3786=ORIENTED_EDGE('',*,*,#2606,.F.);
#3787=ORIENTED_EDGE('',*,*,#2614,.F.);
#3788=ORIENTED_EDGE('',*,*,#2599,.F.);
#3789=ORIENTED_EDGE('',*,*,#2585,.F.);
#3790=ORIENTED_EDGE('',*,*,#2594,.T.);
#3791=ORIENTED_EDGE('',*,*,#2621,.T.);
#3792=ORIENTED_EDGE('',*,*,#2622,.T.);
#3793=ORIENTED_EDGE('',*,*,#2593,.T.);
#3794=ORIENTED_EDGE('',*,*,#2623,.T.);
#3795=ORIENTED_EDGE('',*,*,#2619,.T.);
#3796=ORIENTED_EDGE('',*,*,#2621,.F.);
#3797=ORIENTED_EDGE('',*,*,#2623,.F.);
#3798=ORIENTED_EDGE('',*,*,#2624,.T.);
#3799=ORIENTED_EDGE('',*,*,#2616,.T.);
#3800=ORIENTED_EDGE('',*,*,#2624,.F.);
#3801=ORIENTED_EDGE('',*,*,#2592,.T.);
#3802=ORIENTED_EDGE('',*,*,#2625,.F.);
#3803=ORIENTED_EDGE('',*,*,#2626,.T.);
#3804=ORIENTED_EDGE('',*,*,#2596,.F.);
#3805=ORIENTED_EDGE('',*,*,#2627,.T.);
#3806=ORIENTED_EDGE('',*,*,#2625,.T.);
#3807=ORIENTED_EDGE('',*,*,#2620,.F.);
#3808=ORIENTED_EDGE('',*,*,#2628,.T.);
#3809=ORIENTED_EDGE('',*,*,#2627,.F.);
#3810=ORIENTED_EDGE('',*,*,#2598,.T.);
#3811=ORIENTED_EDGE('',*,*,#2626,.F.);
#3812=ORIENTED_EDGE('',*,*,#2628,.F.);
#3813=ORIENTED_EDGE('',*,*,#2612,.F.);
#3814=ORIENTED_EDGE('',*,*,#2617,.F.);
#3815=ORIENTED_EDGE('',*,*,#2569,.F.);
#3816=ORIENTED_EDGE('',*,*,#2603,.T.);
#3817=ORIENTED_EDGE('',*,*,#2629,.F.);
#3818=ORIENTED_EDGE('',*,*,#2630,.F.);
#3819=ORIENTED_EDGE('',*,*,#2631,.F.);
#3820=ORIENTED_EDGE('',*,*,#2589,.F.);
#3821=ORIENTED_EDGE('',*,*,#2631,.T.);
#3822=ORIENTED_EDGE('',*,*,#2632,.F.);
#3823=ORIENTED_EDGE('',*,*,#2633,.F.);
#3824=ORIENTED_EDGE('',*,*,#2630,.T.);
#3825=ORIENTED_EDGE('',*,*,#2634,.F.);
#3826=ORIENTED_EDGE('',*,*,#2635,.F.);
#3827=ORIENTED_EDGE('',*,*,#2632,.T.);
#3828=ORIENTED_EDGE('',*,*,#2629,.T.);
#3829=ORIENTED_EDGE('',*,*,#2602,.F.);
#3830=ORIENTED_EDGE('',*,*,#2636,.F.);
#3831=ORIENTED_EDGE('',*,*,#2634,.T.);
#3832=ORIENTED_EDGE('',*,*,#2573,.F.);
#3833=ORIENTED_EDGE('',*,*,#2633,.T.);
#3834=ORIENTED_EDGE('',*,*,#2635,.T.);
#3835=ORIENTED_EDGE('',*,*,#2636,.T.);
#3836=ORIENTED_EDGE('',*,*,#2601,.F.);
#3837=ORIENTED_EDGE('',*,*,#2582,.F.);
#3838=ORIENTED_EDGE('',*,*,#2622,.F.);
#3839=ORIENTED_EDGE('',*,*,#2618,.T.);
#3840=ORIENTED_EDGE('',*,*,#2610,.F.);
#3921=CYLINDRICAL_SURFACE('',#4614,0.5);
#3922=CYLINDRICAL_SURFACE('',#4617,0.5);
#3923=CYLINDRICAL_SURFACE('',#4620,0.5);
#3924=CYLINDRICAL_SURFACE('',#4621,0.5);
#3925=CYLINDRICAL_SURFACE('',#4628,61.8868723549169);
#3926=CYLINDRICAL_SURFACE('',#4641,1.);
#3927=CYLINDRICAL_SURFACE('',#4652,1.);
#3928=CYLINDRICAL_SURFACE('',#4656,1.);
#3929=CYLINDRICAL_SURFACE('',#4660,62.3332952479768);
#3930=CYLINDRICAL_SURFACE('',#4664,19.7866355153418);
#4123=ADVANCED_FACE('',(#588),#62,.F.);
#4124=ADVANCED_FACE('',(#589),#63,.F.);
#4125=ADVANCED_FACE('',(#590),#3921,.T.);
#4126=ADVANCED_FACE('',(#591),#64,.F.);
#4127=ADVANCED_FACE('',(#592),#3922,.T.);
#4128=ADVANCED_FACE('',(#593),#65,.F.);
#4129=ADVANCED_FACE('',(#594),#3923,.T.);
#4130=ADVANCED_FACE('',(#595),#3924,.T.);
#4131=ADVANCED_FACE('',(#596),#389,.F.);
#4132=ADVANCED_FACE('',(#597),#225,.T.);
#4133=ADVANCED_FACE('',(#598),#3925,.F.);
#4134=ADVANCED_FACE('',(#599),#226,.T.);
#4135=ADVANCED_FACE('',(#600),#390,.T.);
#4136=ADVANCED_FACE('',(#601),#66,.F.);
#4137=ADVANCED_FACE('',(#602),#47,.T.);
#4138=ADVANCED_FACE('',(#603),#227,.T.);
#4139=ADVANCED_FACE('',(#604),#3926,.T.);
#4140=ADVANCED_FACE('',(#605),#67,.F.);
#4141=ADVANCED_FACE('',(#606),#68,.T.);
#4142=ADVANCED_FACE('',(#607),#48,.T.);
#4143=ADVANCED_FACE('',(#608),#391,.T.);
#4144=ADVANCED_FACE('',(#609),#228,.T.);
#4145=ADVANCED_FACE('',(#610),#69,.F.);
#4146=ADVANCED_FACE('',(#611),#49,.T.);
#4147=ADVANCED_FACE('',(#612),#3927,.T.);
#4148=ADVANCED_FACE('',(#613),#50,.T.);
#4149=ADVANCED_FACE('',(#614),#3928,.T.);
#4150=ADVANCED_FACE('',(#615),#392,.T.);
#4151=ADVANCED_FACE('',(#616),#393,.T.);
#4152=ADVANCED_FACE('',(#617),#3929,.T.);
#4153=ADVANCED_FACE('',(#618),#394,.T.);
#4154=ADVANCED_FACE('',(#619),#70,.T.);
#4155=ADVANCED_FACE('',(#620),#395,.F.);
#4156=ADVANCED_FACE('',(#621),#3930,.T.);
#4165=CLOSED_SHELL('',(#4123,#4124,#4125,#4126,#4127,#4128,#4129,#4130,
#4131,#4132,#4133,#4134,#4135,#4136,#4137,#4138,#4139,#4140,#4141,#4142,
#4143,#4144,#4145,#4146,#4147,#4148,#4149,#4150,#4151,#4152,#4153,#4154,
#4155,#4156));
#4607=AXIS2_PLACEMENT_3D('',#22692,#5617,#5618);
#4608=AXIS2_PLACEMENT_3D('',#22731,#5619,#5620);
#4609=AXIS2_PLACEMENT_3D('',#22774,#5621,#5622);
#4610=AXIS2_PLACEMENT_3D('',#22782,#5623,#5624);
#4611=AXIS2_PLACEMENT_3D('',#22821,#5625,#5626);
#4612=AXIS2_PLACEMENT_3D('',#22864,#5627,#5628);
#4613=AXIS2_PLACEMENT_3D('',#22866,#5629,#5630);
#4614=AXIS2_PLACEMENT_3D('',#22873,#5631,#5632);
#4615=AXIS2_PLACEMENT_3D('',#22876,#5633,#5634);
#4616=AXIS2_PLACEMENT_3D('',#22911,#5637,#5638);
#4617=AXIS2_PLACEMENT_3D('',#22924,#5639,#5640);
#4618=AXIS2_PLACEMENT_3D('',#22927,#5641,#5642);
#4619=AXIS2_PLACEMENT_3D('',#22957,#5645,#5646);
#4620=AXIS2_PLACEMENT_3D('',#22968,#5647,#5648);
#4621=AXIS2_PLACEMENT_3D('',#22971,#5651,#5652);
#4622=AXIS2_PLACEMENT_3D('',#22974,#5655,#5656);
#4623=AXIS2_PLACEMENT_3D('',#22976,#5657,#5658);
#4624=AXIS2_PLACEMENT_3D('',#22990,#5660,#5661);
#4625=AXIS2_PLACEMENT_3D('',#22991,#5662,#5663);
#4626=AXIS2_PLACEMENT_3D('',#22993,#5664,#5665);
#4627=AXIS2_PLACEMENT_3D('',#22994,#5666,#5667);
#4628=AXIS2_PLACEMENT_3D('',#22995,#5668,#5669);
#4629=AXIS2_PLACEMENT_3D('',#22997,#5670,#5671);
#4630=AXIS2_PLACEMENT_3D('',#22999,#5673,#5674);
#4631=AXIS2_PLACEMENT_3D('',#23001,#5675,#5676);
#4632=AXIS2_PLACEMENT_3D('',#23002,#5677,#5678);
#4633=AXIS2_PLACEMENT_3D('',#23003,#5679,#5680);
#4634=AXIS2_PLACEMENT_3D('',#23076,#5684,#5685);
#4635=AXIS2_PLACEMENT_3D('',#23105,#5686,#5687);
#4636=AXIS2_PLACEMENT_3D('',#23107,#5688,#5689);
#4637=AXIS2_PLACEMENT_3D('',#23108,#5690,#5691);
#4638=AXIS2_PLACEMENT_3D('',#23109,#5692,#5693);
#4639=AXIS2_PLACEMENT_3D('',#23110,#5694,#5695);
#4640=AXIS2_PLACEMENT_3D('',#23111,#5696,#5697);
#4641=AXIS2_PLACEMENT_3D('',#23112,#5698,#5699);
#4642=AXIS2_PLACEMENT_3D('',#23115,#5701,#5702);
#4643=AXIS2_PLACEMENT_3D('',#23130,#5705,#5706);
#4644=AXIS2_PLACEMENT_3D('',#23193,#5709,#5710);
#4645=AXIS2_PLACEMENT_3D('',#23194,#5711,#5712);
#4646=AXIS2_PLACEMENT_3D('',#23195,#5713,#5714);
#4647=AXIS2_PLACEMENT_3D('',#23196,#5715,#5716);
#4648=AXIS2_PLACEMENT_3D('',#23213,#5717,#5718);
#4649=AXIS2_PLACEMENT_3D('',#23264,#5719,#5720);
#4650=AXIS2_PLACEMENT_3D('',#23265,#5721,#5722);
#4651=AXIS2_PLACEMENT_3D('',#23266,#5723,#5724);
#4652=AXIS2_PLACEMENT_3D('',#23267,#5725,#5726);
#4653=AXIS2_PLACEMENT_3D('',#23269,#5727,#5728);
#4654=AXIS2_PLACEMENT_3D('',#23271,#5730,#5731);
#4655=AXIS2_PLACEMENT_3D('',#23272,#5732,#5733);
#4656=AXIS2_PLACEMENT_3D('',#23273,#5734,#5735);
#4657=AXIS2_PLACEMENT_3D('',#23275,#5737,#5738);
#4658=AXIS2_PLACEMENT_3D('',#23276,#5739,#5740);
#4659=AXIS2_PLACEMENT_3D('',#23437,#5742,#5743);
#4660=AXIS2_PLACEMENT_3D('',#23438,#5744,#5745);
#4661=AXIS2_PLACEMENT_3D('',#23441,#5747,#5748);
#4662=AXIS2_PLACEMENT_3D('',#23442,#5749,#5750);
#4663=AXIS2_PLACEMENT_3D('',#23545,#5753,#5754);
#4664=AXIS2_PLACEMENT_3D('',#23546,#5755,#5756);
#5617=DIRECTION('axis',(0.,0.,1.));
#5618=DIRECTION('refdir',(1.,0.,0.));
#5619=DIRECTION('center_axis',(0.,1.,0.));
#5620=DIRECTION('ref_axis',(-0.940813565885044,0.,-0.338924525885436));
#5621=DIRECTION('center_axis',(-0.338924525885436,8.35610306180218E-15,
0.940813565885044));
#5622=DIRECTION('ref_axis',(2.13510934712592E-31,1.,-8.88178419700125E-15));
#5623=DIRECTION('center_axis',(0.,1.,0.));
#5624=DIRECTION('ref_axis',(-0.0570391179197161,0.,0.998371944230676));
#5625=DIRECTION('center_axis',(-0.338924525885436,-8.35610306180218E-15,
0.940813565885044));
#5626=DIRECTION('ref_axis',(-0.940813565885044,-4.28735023454931E-31,-0.338924525885436));
#5627=DIRECTION('center_axis',(0.,-1.,0.));
#5628=DIRECTION('ref_axis',(0.0203769416068415,0.,0.99979236856997));
#5629=DIRECTION('center_axis',(0.,-1.,0.));
#5630=DIRECTION('ref_axis',(0.0570391179197162,0.,-0.998371944230676));
#5631=DIRECTION('center_axis',(0.338924525885434,0.,-0.940813565885045));
#5632=DIRECTION('ref_axis',(-0.66525565226961,-0.70710678118655,-0.239655830564025));
#5633=DIRECTION('center_axis',(-0.338924525885432,0.,0.940813565885046));
#5634=DIRECTION('ref_axis',(-0.940813565885046,0.,-0.338924525885432));
#5635=DIRECTION('',(-0.338924525885434,0.,0.940813565885045));
#5636=DIRECTION('',(0.338924525885434,0.,-0.940813565885045));
#5637=DIRECTION('center_axis',(0.,-1.,0.));
#5638=DIRECTION('ref_axis',(-0.940813565885045,0.,-0.338924525885434));
#5639=DIRECTION('center_axis',(0.,-1.,0.));
#5640=DIRECTION('ref_axis',(-0.555722380368519,0.,-0.83136793055635));
#5641=DIRECTION('center_axis',(0.,-1.,0.));
#5642=DIRECTION('ref_axis',(-0.940813565885044,0.,-0.338924525885436));
#5643=DIRECTION('',(0.,-1.,0.));
#5644=DIRECTION('',(0.,1.,0.));
#5645=DIRECTION('center_axis',(0.338924525885437,-2.61128220681318E-15,
-0.940813565885044));
#5646=DIRECTION('ref_axis',(-0.940813565885044,4.44089209850066E-15,-0.338924525885437));
#5647=DIRECTION('center_axis',(0.338924525885434,0.,-0.940813565885045));
#5648=DIRECTION('ref_axis',(-0.665255652269609,0.707106781186551,-0.239655830564025));
#5649=DIRECTION('',(-0.338924525885434,0.,0.940813565885045));
#5650=DIRECTION('',(0.338924525885434,0.,-0.940813565885045));
#5651=DIRECTION('center_axis',(0.,1.,0.));
#5652=DIRECTION('ref_axis',(-0.812306361973871,0.,0.583230978512608));
#5653=DIRECTION('',(0.,-1.,0.));
#5654=DIRECTION('',(0.,1.,0.));
#5655=DIRECTION('center_axis',(0.,-1.,0.));
#5656=DIRECTION('ref_axis',(1.,0.,0.));
#5657=DIRECTION('center_axis',(0.,1.,0.));
#5658=DIRECTION('ref_axis',(0.141943234522443,0.,-0.989874799241453));
#5659=DIRECTION('',(4.67836035237689E-14,0.,1.));
#5660=DIRECTION('center_axis',(0.,-1.,0.));
#5661=DIRECTION('ref_axis',(0.335988807373518,0.,-0.941865978427781));
#5662=DIRECTION('center_axis',(0.,1.,0.));
#5663=DIRECTION('ref_axis',(0.147769932247684,0.,-0.989021762714813));
#5664=DIRECTION('center_axis',(0.,-1.,0.));
#5665=DIRECTION('ref_axis',(0.141943234522443,0.,-0.989874799241453));
#5666=DIRECTION('center_axis',(-0.950173445040706,-4.15296743349361E-15,
-0.31172170976606));
#5667=DIRECTION('ref_axis',(-0.31172170976606,-2.25212199954037E-32,0.950173445040706));
#5668=DIRECTION('center_axis',(0.,-1.,0.));
#5669=DIRECTION('ref_axis',(-0.032150446799728,0.,-0.999483040761862));
#5670=DIRECTION('center_axis',(0.,1.,0.));
#5671=DIRECTION('ref_axis',(0.141943234522443,0.,-0.989874799241453));
#5672=DIRECTION('',(0.,-1.,0.));
#5673=DIRECTION('center_axis',(0.,1.,0.));
#5674=DIRECTION('ref_axis',(0.147769932247684,0.,-0.989021762714813));
#5675=DIRECTION('center_axis',(0.,-1.,0.));
#5676=DIRECTION('ref_axis',(0.141943234522443,0.,-0.989874799241453));
#5677=DIRECTION('center_axis',(-0.950173445040706,1.3843224778312E-15,-0.31172170976606));
#5678=DIRECTION('ref_axis',(2.67362611073496E-30,-1.,-4.44089209850063E-15));
#5679=DIRECTION('center_axis',(-0.940813565885045,0.,-0.338924525885434));
#5680=DIRECTION('ref_axis',(0.338924525885434,0.,-0.940813565885045));
#5681=DIRECTION('',(0.338924525885434,0.,-0.940813565885045));
#5682=DIRECTION('',(0.,1.,0.));
#5683=DIRECTION('',(0.338924525885434,0.,-0.940813565885045));
#5684=DIRECTION('center_axis',(-0.944875085787754,-5.26189473139136E-12,
-0.327431019082774));
#5685=DIRECTION('ref_axis',(0.327431019082774,4.11381421934135E-29,-0.944875085787754));
#5686=DIRECTION('center_axis',(0.,0.,1.));
#5687=DIRECTION('ref_axis',(1.,0.,0.));
#5688=DIRECTION('center_axis',(0.,-1.,0.));
#5689=DIRECTION('ref_axis',(1.,0.,-4.66293670342563E-14));
#5690=DIRECTION('center_axis',(-4.67836035237689E-14,0.,-1.));
#5691=DIRECTION('ref_axis',(0.707106781186546,-0.707106781186549,-3.30810032999998E-14));
#5692=DIRECTION('center_axis',(0.,-1.,0.));
#5693=DIRECTION('ref_axis',(0.,0.,-1.));
#5694=DIRECTION('center_axis',(0.,-1.,0.));
#5695=DIRECTION('ref_axis',(0.335988807373518,0.,-0.941865978427781));
#5696=DIRECTION('center_axis',(0.,1.,0.));
#5697=DIRECTION('ref_axis',(0.335988807373518,0.,-0.941865978427781));
#5698=DIRECTION('center_axis',(4.67836035237689E-14,0.,1.));
#5699=DIRECTION('ref_axis',(0.707106781186546,-0.707106781186549,-3.30810032999998E-14));
#5700=DIRECTION('',(4.67836035237689E-14,0.,1.));
#5701=DIRECTION('center_axis',(4.67836035237689E-14,0.,1.));
#5702=DIRECTION('ref_axis',(0.707106781186546,-0.707106781186549,-3.30810032999998E-14));
#5703=DIRECTION('',(-4.67836035237689E-14,0.,-1.));
#5704=DIRECTION('',(0.,1.,0.));
#5705=DIRECTION('center_axis',(0.,1.,0.));
#5706=DIRECTION('ref_axis',(1.,0.,-4.66293670342563E-14));
#5707=DIRECTION('',(0.,-1.,0.));
#5708=DIRECTION('',(0.,-1.,0.));
#5709=DIRECTION('center_axis',(-0.894799777334527,-0.323660756971229,0.307533856475823));
#5710=DIRECTION('ref_axis',(0.446467645504215,-0.648673148404086,0.616352000124485));
#5711=DIRECTION('center_axis',(0.,-1.,0.));
#5712=DIRECTION('ref_axis',(0.586633740179502,0.,0.809852366103235));
#5713=DIRECTION('center_axis',(0.,-1.,0.));
#5714=DIRECTION('ref_axis',(1.,0.,0.));
#5715=DIRECTION('center_axis',(0.,-1.,0.));
#5716=DIRECTION('ref_axis',(0.,0.,-1.));
#5717=DIRECTION('center_axis',(0.,1.,0.));
#5718=DIRECTION('ref_axis',(0.335988807373518,0.,-0.941865978427781));
#5719=DIRECTION('center_axis',(-0.944875085789614,0.,-0.327431019077409));
#5720=DIRECTION('ref_axis',(0.,1.,0.));
#5721=DIRECTION('center_axis',(0.,0.,1.));
#5722=DIRECTION('ref_axis',(1.,0.,0.));
#5723=DIRECTION('center_axis',(-4.67836035237689E-14,0.,-1.));
#5724=DIRECTION('ref_axis',(0.707106781186546,0.707106781186549,-3.30810032999998E-14));
#5725=DIRECTION('center_axis',(4.67836035237689E-14,0.,1.));
#5726=DIRECTION('ref_axis',(0.707106781186546,0.707106781186549,-3.30810032999998E-14));
#5727=DIRECTION('center_axis',(4.67836035237689E-14,0.,1.));
#5728=DIRECTION('ref_axis',(0.707106781186546,0.707106781186549,-3.30810032999998E-14));
#5729=DIRECTION('',(-4.67836035237689E-14,0.,-1.));
#5730=DIRECTION('center_axis',(-0.894799777334522,0.323660756971238,0.307533856475827));
#5731=DIRECTION('ref_axis',(0.446467645504229,0.648673148404085,0.616352000124476));
#5732=DIRECTION('center_axis',(0.,1.,0.));
#5733=DIRECTION('ref_axis',(0.586633740179502,0.,0.809852366103235));
#5734=DIRECTION('center_axis',(0.,-1.,0.));
#5735=DIRECTION('ref_axis',(0.586633740179504,0.,0.809852366103234));
#5736=DIRECTION('',(0.,1.,0.));
#5737=DIRECTION('center_axis',(1.,0.,-4.67836035237689E-14));
#5738=DIRECTION('ref_axis',(4.67836035237689E-14,0.,1.));
#5739=DIRECTION('center_axis',(0.,-1.,0.));
#5740=DIRECTION('ref_axis',(1.,0.,0.));
#5741=DIRECTION('',(-4.18364780870191E-14,0.,-1.));
#5742=DIRECTION('center_axis',(0.,-1.,0.));
#5743=DIRECTION('ref_axis',(-0.032150677597388,0.,-0.999483033337749));
#5744=DIRECTION('center_axis',(0.,1.,0.));
#5745=DIRECTION('ref_axis',(-0.032150677597388,0.,-0.999483033337749));
#5746=DIRECTION('',(0.,1.,0.));
#5747=DIRECTION('center_axis',(0.,-1.,0.));
#5748=DIRECTION('ref_axis',(-0.032150677597388,0.,-0.999483033337749));
#5749=DIRECTION('center_axis',(-1.,0.,4.18364780870191E-14));
#5750=DIRECTION('ref_axis',(4.18364780870191E-14,0.,1.));
#5751=DIRECTION('',(0.,1.,0.));
#5752=DIRECTION('',(-4.18364780870191E-14,0.,-1.));
#5753=DIRECTION('center_axis',(0.,-1.,0.));
#5754=DIRECTION('ref_axis',(1.,0.,0.));
#5755=DIRECTION('center_axis',(0.,-1.,0.));
#5756=DIRECTION('ref_axis',(0.0278513911097204,0.,-0.999612074763632));
#22692=CARTESIAN_POINT('',(0.,0.,0.));
#22693=CARTESIAN_POINT('Ctrl Pts',(46.6861496741435,4.13165936500604,6.75210248110235));
#22694=CARTESIAN_POINT('Ctrl Pts',(46.6467382040187,4.13173032837167,6.8615039640666));
#22695=CARTESIAN_POINT('Ctrl Pts',(46.5809898678815,4.07139842264618,7.04401340746142));
#22696=CARTESIAN_POINT('Ctrl Pts',(46.5181050726922,3.86354903122596,7.21857400689702));
#22697=CARTESIAN_POINT('Ctrl Pts',(46.5046271380005,3.70887953224881,7.25598712642546));
#22698=CARTESIAN_POINT('Ctrl Pts',(46.5046469694585,3.63131831090395,7.25593207669225));
#22699=CARTESIAN_POINT('Ctrl Pts',(46.6861648307274,4.2064483703636,6.75206052368169));
#22700=CARTESIAN_POINT('Ctrl Pts',(46.6415880227693,4.2102116935304,6.87576092573886));
#22701=CARTESIAN_POINT('Ctrl Pts',(46.5658363543261,4.14848673640705,7.0861290861269));
#22702=CARTESIAN_POINT('Ctrl Pts',(46.4900735883089,3.90919827275704,7.29633200080862));
#22703=CARTESIAN_POINT('Ctrl Pts',(46.4733614735456,3.72414766997645,7.34277691560461));
#22704=CARTESIAN_POINT('Ctrl Pts',(46.4733860630999,3.63125085693363,7.34270857847526));
#22705=CARTESIAN_POINT('Ctrl Pts',(46.7183800447354,4.35575113079639,6.76357123269517));
#22706=CARTESIAN_POINT('Ctrl Pts',(46.6667328898876,4.36685422640062,6.91699804310752));
#22707=CARTESIAN_POINT('Ctrl Pts',(46.5768274780168,4.30231304999428,7.18491601275544));
#22708=CARTESIAN_POINT('Ctrl Pts',(46.4820223126629,4.00023029397859,7.46856355573902));
#22709=CARTESIAN_POINT('Ctrl Pts',(46.4603525972319,3.75460132906098,7.53347058371532));
#22710=CARTESIAN_POINT('Ctrl Pts',(46.460384480148,3.63111631405149,7.53337508531403));
#22711=CARTESIAN_POINT('Ctrl Pts',(46.8757561668702,4.56603451100179,6.82013223242444));
#22712=CARTESIAN_POINT('Ctrl Pts',(46.8243018044365,4.58250926196892,7.01900975145347));
#22713=CARTESIAN_POINT('Ctrl Pts',(46.7343292407208,4.5031002935665,7.36952281620736));
#22714=CARTESIAN_POINT('Ctrl Pts',(46.638383000099,4.1127406122417,7.74468925829955));
#22715=CARTESIAN_POINT('Ctrl Pts',(46.616220839815,3.7921233777235,7.83123568433033));
#22716=CARTESIAN_POINT('Ctrl Pts',(46.6162534469586,3.63095054220852,7.83110834859193));
#22717=CARTESIAN_POINT('Ctrl Pts',(47.0510239491272,4.63163976411415,6.88322984349305));
#22718=CARTESIAN_POINT('Ctrl Pts',(47.0082783943361,4.64056070504751,7.09954757890675));
#22719=CARTESIAN_POINT('Ctrl Pts',(46.9358664296334,4.53765652876905,7.46970543244382));
#22720=CARTESIAN_POINT('Ctrl Pts',(46.8630216802537,4.12014583132121,7.84521978438382));
#22721=CARTESIAN_POINT('Ctrl Pts',(46.8469158520526,3.79451524716846,7.92824101697815));
#22722=CARTESIAN_POINT('Ctrl Pts',(46.8469395494882,3.63093997420058,7.92811886303569));
#22723=CARTESIAN_POINT('Ctrl Pts',(47.1565761357334,4.63165926631602,6.92125495912786));
#22724=CARTESIAN_POINT('Ctrl Pts',(47.1190493074978,4.63179909627843,7.13934266665166));
#22725=CARTESIAN_POINT('Ctrl Pts',(47.0568496727956,4.51113104304455,7.50308186089014));
#22726=CARTESIAN_POINT('Ctrl Pts',(46.9978527681235,4.09543269263203,7.85086983906624));
#22727=CARTESIAN_POINT('Ctrl Pts',(46.985256719747,3.78609758552286,7.92539939233487));
#22728=CARTESIAN_POINT('Ctrl Pts',(46.9852752536658,3.63097716158626,7.92528972939672));
#22729=CARTESIAN_POINT('',(46.4793862705605,3.63165946910083,7.4910739147271));
#22730=CARTESIAN_POINT('',(46.9852421795911,3.63165946910083,7.92529064498531));
#22731=CARTESIAN_POINT('Origin',(46.9750537087877,3.63165946910083,7.42539446070033));
#22732=CARTESIAN_POINT('',(47.1564408307335,4.63165946910083,6.92188570884001));
#22733=CARTESIAN_POINT('Ctrl Pts',(46.9852421795911,3.63165946910083,7.92529064498533));
#22734=CARTESIAN_POINT('Ctrl Pts',(46.9852421795911,3.67152847702579,7.92529064498533));
#22735=CARTESIAN_POINT('Ctrl Pts',(46.9856617576314,3.71139629383976,7.92289294206818));
#22736=CARTESIAN_POINT('Ctrl Pts',(46.9864809263889,3.75094114378544,7.91812438514576));
#22737=CARTESIAN_POINT('Ctrl Pts',(46.987300394655,3.79050045231676,7.91335408471972));
#22738=CARTESIAN_POINT('Ctrl Pts',(46.9885197537897,3.82973593634109,7.90621131868988));
#22739=CARTESIAN_POINT('Ctrl Pts',(46.990120623989,3.86833498313616,7.8967743079273));
#22740=CARTESIAN_POINT('Ctrl Pts',(46.991725286537,3.90702546835329,7.88731494155118));
#22741=CARTESIAN_POINT('Ctrl Pts',(46.9937132815878,3.94507590371365,7.87555067389803));
#22742=CARTESIAN_POINT('Ctrl Pts',(46.9960675879378,3.98219017156174,7.86160926054568));
#22743=CARTESIAN_POINT('Ctrl Pts',(46.9981383536307,4.01483458615883,7.84934687995914));
#22744=CARTESIAN_POINT('Ctrl Pts',(47.0004925394058,4.04675480199022,7.83540106098309));
#22745=CARTESIAN_POINT('Ctrl Pts',(47.0031193862113,4.07776647838611,7.81988733921945));
#22746=CARTESIAN_POINT('Ctrl Pts',(47.0063554421103,4.11597027395028,7.80077572954276));
#22747=CARTESIAN_POINT('Ctrl Pts',(47.0100043369411,4.15281712248742,7.77927345884883));
#22748=CARTESIAN_POINT('Ctrl Pts',(47.0140201692982,4.18802664862582,7.75561393361822));
#22749=CARTESIAN_POINT('Ctrl Pts',(47.0180513055259,4.22337035417768,7.73186424468573));
#22750=CARTESIAN_POINT('Ctrl Pts',(47.0224522066382,4.25706392790331,7.70594127813406));
#22751=CARTESIAN_POINT('Ctrl Pts',(47.0271771428546,4.28886502022712,7.67811395812653));
#22752=CARTESIAN_POINT('Ctrl Pts',(47.0319338280211,4.32087979824855,7.65009965396675));
#22753=CARTESIAN_POINT('Ctrl Pts',(47.0370189428221,4.35097632510684,7.62015580277312));
#22754=CARTESIAN_POINT('Ctrl Pts',(47.0423861535344,4.37895330700274,7.58858295363978));
#22755=CARTESIAN_POINT('Ctrl Pts',(47.0453675812267,4.39449421885468,7.5710445763008));
#22756=CARTESIAN_POINT('Ctrl Pts',(47.0484360582723,4.40938194656237,7.55300396459847));
#22757=CARTESIAN_POINT('Ctrl Pts',(47.051583642697,4.42358842273374,7.53451522576715));
#22758=CARTESIAN_POINT('Ctrl Pts',(47.0581899359112,4.45340562045305,7.49571022059454));
#22759=CARTESIAN_POINT('Ctrl Pts',(47.065142388108,4.48023980475269,7.4549047021496));
#22760=CARTESIAN_POINT('Ctrl Pts',(47.0723688007126,4.50391212229452,7.41254059878685));
#22761=CARTESIAN_POINT('Ctrl Pts',(47.0798141341055,4.52830158161893,7.36889309473683));
#22762=CARTESIAN_POINT('Ctrl Pts',(47.087550305732,4.54933477550803,7.3235912995658));
#22763=CARTESIAN_POINT('Ctrl Pts',(47.095497140004,4.56687155697433,7.27711929567226));
#22764=CARTESIAN_POINT('Ctrl Pts',(47.1035574048721,4.58465865290626,7.22998396511051));
#22765=CARTESIAN_POINT('Ctrl Pts',(47.111834408255,4.59884897342125,7.18164485798867));
#22766=CARTESIAN_POINT('Ctrl Pts',(47.1202429072472,4.60935039329557,7.132606053074));
#22767=CARTESIAN_POINT('Ctrl Pts',(47.1287650304598,4.61999371907335,7.08290458577658));
#22768=CARTESIAN_POINT('Ctrl Pts',(47.1374222396982,4.62684784892612,7.03248439243499));
#22769=CARTESIAN_POINT('Ctrl Pts',(47.1461239307463,4.62987020526441,6.98186857301297));
#22770=CARTESIAN_POINT('Ctrl Pts',(47.1495578751189,4.63106291636878,6.96189407526204));
#22771=CARTESIAN_POINT('Ctrl Pts',(47.1529987256109,4.63165946910083,6.94188909356262));
#22772=CARTESIAN_POINT('Ctrl Pts',(47.1564408307335,4.63165946910083,6.92188570884));
#22773=CARTESIAN_POINT('',(46.686034047791,4.13165946910083,6.7524234458973));
#22774=CARTESIAN_POINT('Origin',(47.1564408307335,4.13165946910083,6.92188570884002));
#22775=CARTESIAN_POINT('',(46.5046469258452,3.63165946910083,7.25593219775761));
#22776=CARTESIAN_POINT('Ctrl Pts',(46.686034047791,4.13165946910083,6.7524234458973));
#22777=CARTESIAN_POINT('Ctrl Pts',(46.6466610234604,4.13165946910083,6.86171820797849));
#22778=CARTESIAN_POINT('Ctrl Pts',(46.5809635080922,4.07131129719481,7.04408657905414));
#22779=CARTESIAN_POINT('Ctrl Pts',(46.5181314324815,3.86363615667733,7.2185008353043));
#22780=CARTESIAN_POINT('Ctrl Pts',(46.5046469258452,3.70910645473421,7.25593219775761));
#22781=CARTESIAN_POINT('Ctrl Pts',(46.5046469258452,3.63165946910083,7.25593219775761));
#22782=CARTESIAN_POINT('Origin',(46.8597130365341,3.63165946910083,7.41851908154457));
#22783=CARTESIAN_POINT('Ctrl Pts',(46.5046473528159,-3.63059149855109,7.25593101253869));
#22784=CARTESIAN_POINT('Ctrl Pts',(46.5045851322103,-3.70839938355921,7.25610372942774));
#22785=CARTESIAN_POINT('Ctrl Pts',(46.5146795236394,-3.82415536695909,7.228082917505));
#22786=CARTESIAN_POINT('Ctrl Pts',(46.5678509837999,-4.04941234271178,7.08048536342935));
#22787=CARTESIAN_POINT('Ctrl Pts',(46.6337785675335,-4.1319627243891,6.89747835034739));
#22788=CARTESIAN_POINT('Ctrl Pts',(46.6863959957155,-4.13165842258026,6.75141872215656));
#22789=CARTESIAN_POINT('Ctrl Pts',(46.4733865349565,-3.6303803307724,7.34270726672911));
#22790=CARTESIAN_POINT('Ctrl Pts',(46.4733098915423,-3.72357375245234,7.34292032668699));
#22791=CARTESIAN_POINT('Ctrl Pts',(46.4857448581586,-3.86198192710135,7.30835231108237));
#22792=CARTESIAN_POINT('Ctrl Pts',(46.5502018222126,-4.12463364349051,7.12951212492674));
#22793=CARTESIAN_POINT('Ctrl Pts',(46.6269356550349,-4.21168567686206,6.91642084451281));
#22794=CARTESIAN_POINT('Ctrl Pts',(46.6864434208004,-4.20642428381315,6.75128743826182));
#22795=CARTESIAN_POINT('Ctrl Pts',(46.4603850872009,-3.62995913755521,7.5333732676333));
#22796=CARTESIAN_POINT('Ctrl Pts',(46.4602864022167,-3.75384045282994,7.53366876770548));
#22797=CARTESIAN_POINT('Ctrl Pts',(46.4762986367123,-3.93741399174525,7.485722011047));
#22798=CARTESIAN_POINT('Ctrl Pts',(46.557549294366,-4.27471561178946,7.24255755482672));
#22799=CARTESIAN_POINT('Ctrl Pts',(46.6497653146017,-4.37079649213517,6.96740001798986));
#22800=CARTESIAN_POINT('Ctrl Pts',(46.7187027995757,-4.35568103713875,6.7626124413514));
#22801=CARTESIAN_POINT('Ctrl Pts',(46.6162653945892,-3.6294401541011,7.8311275649258));
#22802=CARTESIAN_POINT('Ctrl Pts',(46.6161646216497,-3.79113322873311,7.83152127712809));
#22803=CARTESIAN_POINT('Ctrl Pts',(46.6325160222927,-4.03070572037737,7.76763770947141));
#22804=CARTESIAN_POINT('Ctrl Pts',(46.7149034765713,-4.46813006456083,7.44558925601383));
#22805=CARTESIAN_POINT('Ctrl Pts',(46.8074107262328,-4.588317987608,7.08433941933847));
#22806=CARTESIAN_POINT('Ctrl Pts',(46.8760891498065,-4.56594592129301,6.81889353011202));
#22807=CARTESIAN_POINT('Ctrl Pts',(46.8469869465433,-3.62940711399243,7.92813626289466));
#22808=CARTESIAN_POINT('Ctrl Pts',(46.8469132135861,-3.79350638218252,7.92851633731934));
#22809=CARTESIAN_POINT('Ctrl Pts',(46.8588759569925,-4.03697057004181,7.86685151402129));
#22810=CARTESIAN_POINT('Ctrl Pts',(46.9209122979257,-4.49671412053998,7.5470074194169));
#22811=CARTESIAN_POINT('Ctrl Pts',(46.9942655102648,-4.64391672140692,7.17065803186552));
#22812=CARTESIAN_POINT('Ctrl Pts',(47.0513267498103,-4.63159638131279,6.88189077518217));
#22813=CARTESIAN_POINT('Ctrl Pts',(46.9853459842389,-3.62952361504528,7.92528616511393));
#22814=CARTESIAN_POINT('Ctrl Pts',(46.9852878014976,-3.78513304186471,7.92563022056898));
#22815=CARTESIAN_POINT('Ctrl Pts',(46.9947270293396,-4.01663607192479,7.86981222866872));
#22816=CARTESIAN_POINT('Ctrl Pts',(47.0445674957162,-4.46714312456898,7.57576607873376));
#22817=CARTESIAN_POINT('Ctrl Pts',(47.1067651506559,-4.63225727414747,7.21107711520724));
#22818=CARTESIAN_POINT('Ctrl Pts',(47.1568643602425,-4.63165742900804,6.91991124874024));
#22819=CARTESIAN_POINT('',(46.686034047791,-4.13165946910082,6.7524234458973));
#22820=CARTESIAN_POINT('',(47.1564408307335,-4.63165946910082,6.92188570884001));
#22821=CARTESIAN_POINT('Origin',(47.1564408307335,-4.13165946910082,6.92188570884002));
#22822=CARTESIAN_POINT('',(46.9852421795911,-3.63165946910083,7.92529064498531));
#22823=CARTESIAN_POINT('Ctrl Pts',(47.1564408307335,-4.63165946910083,6.92188570884));
#22824=CARTESIAN_POINT('Ctrl Pts',(47.1480140170322,-4.63165946910083,6.97085713488546));
#22825=CARTESIAN_POINT('Ctrl Pts',(47.1395935372251,-4.62808037647553,7.01986113496256));
#22826=CARTESIAN_POINT('Ctrl Pts',(47.131262570954,-4.62093455138398,7.06841459938196));
#22827=CARTESIAN_POINT('Ctrl Pts',(47.1229974613597,-4.613845214373,7.116584246401));
#22828=CARTESIAN_POINT('Ctrl Pts',(47.1148204463948,-4.60324526052124,7.16431030846801));
#22829=CARTESIAN_POINT('Ctrl Pts',(47.1068110838378,-4.58919780885303,7.21111906483794));
#22830=CARTESIAN_POINT('Ctrl Pts',(47.0988591605656,-4.57525109873224,7.25759213138594));
#22831=CARTESIAN_POINT('Ctrl Pts',(47.0910724786717,-4.5579060519702,7.30316082472435));
#22832=CARTESIAN_POINT('Ctrl Pts',(47.0835274294847,-4.53727617799087,7.34736195753565));
#22833=CARTESIAN_POINT('Ctrl Pts',(47.0761627505453,-4.51713947713545,7.39050642801491));
#22834=CARTESIAN_POINT('Ctrl Pts',(47.0690282667772,-4.49387313010114,7.43234773661696));
#22835=CARTESIAN_POINT('Ctrl Pts',(47.0621939029827,-4.46763272108791,7.4724583193628));
#22836=CARTESIAN_POINT('Ctrl Pts',(47.0551084659439,-4.4404283211574,7.51404244001858));
#22837=CARTESIAN_POINT('Ctrl Pts',(47.0483455830168,-4.41002672598321,7.55376596857338));
#22838=CARTESIAN_POINT('Ctrl Pts',(47.0419822780536,-4.37666097695831,7.59116030088757));
#22839=CARTESIAN_POINT('Ctrl Pts',(47.0360532053804,-4.34557210853064,7.62600284185342));
#22840=CARTESIAN_POINT('Ctrl Pts',(47.0304710043537,-4.31191022757954,7.65882301129956));
#22841=CARTESIAN_POINT('Ctrl Pts',(47.0252976393728,-4.27591443953535,7.68925240584234));
#22842=CARTESIAN_POINT('Ctrl Pts',(47.0249187534582,-4.27327818689815,7.69148098801738));
#22843=CARTESIAN_POINT('Ctrl Pts',(47.0245420604123,-4.27062943822396,7.69369675255096));
#22844=CARTESIAN_POINT('Ctrl Pts',(47.0241675845705,-4.26796829819623,7.69589955768561));
#22845=CARTESIAN_POINT('Ctrl Pts',(47.0200852466292,-4.23895795442667,7.71991337640538));
#22846=CARTESIAN_POINT('Ctrl Pts',(47.0162689643525,-4.20842353959352,7.74242325255637));
#22847=CARTESIAN_POINT('Ctrl Pts',(47.0127500788317,-4.17657725649026,7.76319358679969));
#22848=CARTESIAN_POINT('Ctrl Pts',(47.0092311933109,-4.144730973387,7.783963921043));
#22849=CARTESIAN_POINT('Ctrl Pts',(47.0060096815111,-4.11157336723279,7.8029941292581));
#22850=CARTESIAN_POINT('Ctrl Pts',(47.0031177369572,-4.07735827430611,7.82009076834584));
#22851=CARTESIAN_POINT('Ctrl Pts',(46.9998935700605,-4.03921260175829,7.83915144422086));
#22852=CARTESIAN_POINT('Ctrl Pts',(46.9970796175557,-3.99976085751644,7.85580659935101));
#22853=CARTESIAN_POINT('Ctrl Pts',(46.9946965256702,-3.95932346117812,7.86988171412677));
#22854=CARTESIAN_POINT('Ctrl Pts',(46.9923191156137,-3.91898247672032,7.88392327065184));
#22855=CARTESIAN_POINT('Ctrl Pts',(46.990370497899,-3.8776609874032,7.8953968044727));
#22856=CARTESIAN_POINT('Ctrl Pts',(46.9888726507954,-3.83570196062553,7.90417444862372));
#22857=CARTESIAN_POINT('Ctrl Pts',(46.9873788593879,-3.79385654561952,7.91292832569099));
#22858=CARTESIAN_POINT('Ctrl Pts',(46.9863333881254,-3.75137753185371,7.91900070201506));
#22859=CARTESIAN_POINT('Ctrl Pts',(46.9857597266497,-3.70862276753427,7.92231341004287));
#22860=CARTESIAN_POINT('Ctrl Pts',(46.9854164778235,-3.6830405674236,7.9242955601266));
#22861=CARTESIAN_POINT('Ctrl Pts',(46.9852421795911,-3.6573599489112,7.92529064498533));
#22862=CARTESIAN_POINT('Ctrl Pts',(46.9852421795911,-3.63165946910083,7.92529064498533));
#22863=CARTESIAN_POINT('',(46.4793862705605,-3.63165946910083,7.49107391472711));
#22864=CARTESIAN_POINT('Origin',(46.9750537087877,-3.63165946910083,7.42539446070033));
#22865=CARTESIAN_POINT('',(46.5046469258452,-3.63165946910083,7.25593219775761));
#22866=CARTESIAN_POINT('Origin',(46.8597130365341,-3.63165946910083,7.41851908154457));
#22867=CARTESIAN_POINT('Ctrl Pts',(46.5046469258452,-3.63165946910083,7.25593219775761));
#22868=CARTESIAN_POINT('Ctrl Pts',(46.5046469258452,-3.70910645473421,7.25593219775761));
#22869=CARTESIAN_POINT('Ctrl Pts',(46.5147491688035,-3.82445041356865,7.22788959093758));
#22870=CARTESIAN_POINT('Ctrl Pts',(46.5677813386358,-4.04911729610222,7.08067868999677));
#22871=CARTESIAN_POINT('Ctrl Pts',(46.6335366820169,-4.13165946910083,6.89814979533889));
#22872=CARTESIAN_POINT('Ctrl Pts',(46.686034047791,-4.13165946910082,6.7524234458973));
#22873=CARTESIAN_POINT('Origin',(47.6576678782476,-4.13165946910082,5.53053993751283));
#22874=CARTESIAN_POINT('',(48.4890896340131,-4.13165946910082,1.74735881939682));
#22875=CARTESIAN_POINT('',(48.9594964169556,-4.63165946910082,1.91682108233953));
#22876=CARTESIAN_POINT('Origin',(48.9594964169556,-4.13165946910082,1.91682108233953));
#22877=CARTESIAN_POINT('',(47.6576678782476,-4.63165946910082,5.53053993751283));
#22878=CARTESIAN_POINT('',(47.187261095305,-4.13165946910082,5.36107767457011));
#22879=CARTESIAN_POINT('Ctrl Pts',(48.4890896340131,-4.13165946910082,1.74735881939682));
#22880=CARTESIAN_POINT('Ctrl Pts',(48.528033400252,-4.13165946910082,1.63925562595442));
#22881=CARTESIAN_POINT('Ctrl Pts',(48.59296896781,-4.0698690772923,1.45900233001064));
#22882=CARTESIAN_POINT('Ctrl Pts',(48.6538411747882,-3.86114173341796,1.29002843247154));
#22883=CARTESIAN_POINT('Ctrl Pts',(48.6666566035268,-3.70826210137736,1.25445434948526));
#22884=CARTESIAN_POINT('Ctrl Pts',(48.6666566035268,-3.63165946910083,1.25445434948526));
#22885=CARTESIAN_POINT('Ctrl Pts',(48.4890896340131,-4.2625591630004,1.74735881939682));
#22886=CARTESIAN_POINT('Ctrl Pts',(48.5374817032876,-4.25698138037902,1.61355961347516));
#22887=CARTESIAN_POINT('Ctrl Pts',(48.6157021694607,-4.17210624395573,1.39606123956507));
#22888=CARTESIAN_POINT('Ctrl Pts',(48.6877387227602,-3.91206590758877,1.19649815595369));
#22889=CARTESIAN_POINT('Ctrl Pts',(48.7025708074101,-3.72526406128552,1.1547608553863));
#22890=CARTESIAN_POINT('Ctrl Pts',(48.7025708074101,-3.63165946910083,1.1547608553863));
#22891=CARTESIAN_POINT('Ctrl Pts',(48.5910979765086,-4.52323379775168,1.78410693865264));
#22892=CARTESIAN_POINT('Ctrl Pts',(48.6485962811641,-4.50700223220463,1.59589909277704));
#22893=CARTESIAN_POINT('Ctrl Pts',(48.7401801263016,-4.37605369011658,1.29919670157222));
#22894=CARTESIAN_POINT('Ctrl Pts',(48.8226835402575,-4.01396661770324,1.03419011377791));
#22895=CARTESIAN_POINT('Ctrl Pts',(48.8399066101512,-3.75914369554963,0.97936619857827));
#22896=CARTESIAN_POINT('Ctrl Pts',(48.8399066101512,-3.63165946910082,0.97936619857827));
#22897=CARTESIAN_POINT('Ctrl Pts',(48.8363442091647,-4.63165946910083,1.87245596564607));
#22898=CARTESIAN_POINT('Ctrl Pts',(48.8847421900004,-4.62278702779619,1.65657705029431));
#22899=CARTESIAN_POINT('Ctrl Pts',(48.9644640517391,-4.48805314820043,1.30657194968926));
#22900=CARTESIAN_POINT('Ctrl Pts',(49.03889631391,-4.07555797544749,0.986222066672633));
#22901=CARTESIAN_POINT('Ctrl Pts',(49.0544843934583,-3.77992147471384,0.919526552336082));
#22902=CARTESIAN_POINT('Ctrl Pts',(49.0544843934583,-3.63165946910083,0.919526552336082));
#22903=CARTESIAN_POINT('Ctrl Pts',(48.9594964169557,-4.63165946910083,1.91682108233953));
#22904=CARTESIAN_POINT('Ctrl Pts',(49.002637914566,-4.63165946910083,1.69928191144716));
#22905=CARTESIAN_POINT('Ctrl Pts',(49.0757300098058,-4.50807868548377,1.33641576134982));
#22906=CARTESIAN_POINT('Ctrl Pts',(49.1455292082179,-4.09062399773509,0.996113990481237));
#22907=CARTESIAN_POINT('Ctrl Pts',(49.160334755135,-3.78486473365389,0.924458462629198));
#22908=CARTESIAN_POINT('Ctrl Pts',(49.160334755135,-3.63165946910083,0.924458462629198));
#22909=CARTESIAN_POINT('',(48.6666566035268,-3.63165946910083,1.25445434948526));
#22910=CARTESIAN_POINT('',(49.160334755135,-3.63165946910083,0.924458462629196));
#22911=CARTESIAN_POINT('Origin',(49.1370633864694,-3.63165946910083,1.42391661242798));
#22912=CARTESIAN_POINT('Ctrl Pts',(49.160334755135,-3.63165946910083,0.924458462629198));
#22913=CARTESIAN_POINT('Ctrl Pts',(49.160334755135,-3.78486473365389,0.924458462629198));
#22914=CARTESIAN_POINT('Ctrl Pts',(49.1455292082179,-4.09062399773509,0.996113990481237));
#22915=CARTESIAN_POINT('Ctrl Pts',(49.0757300098058,-4.50807868548377,1.33641576134982));
#22916=CARTESIAN_POINT('Ctrl Pts',(49.002637914566,-4.63165946910083,1.69928191144716));
#22917=CARTESIAN_POINT('Ctrl Pts',(48.9594964169557,-4.63165946910083,1.91682108233953));
#22918=CARTESIAN_POINT('Ctrl Pts',(48.4890896340131,-4.13165946910082,1.74735881939682));
#22919=CARTESIAN_POINT('Ctrl Pts',(48.528033400252,-4.13165946910082,1.63925562595442));
#22920=CARTESIAN_POINT('Ctrl Pts',(48.59296896781,-4.0698690772923,1.45900233001064));
#22921=CARTESIAN_POINT('Ctrl Pts',(48.6538411747882,-3.86114173341796,1.29002843247154));
#22922=CARTESIAN_POINT('Ctrl Pts',(48.6666566035268,-3.70826210137736,1.25445434948526));
#22923=CARTESIAN_POINT('Ctrl Pts',(48.6666566035268,-3.63165946910083,1.25445434948526));
#22924=CARTESIAN_POINT('Origin',(49.1370633864693,-3.63165946910082,1.42391661242798));
#22925=CARTESIAN_POINT('',(48.6666566035268,3.63165946910083,1.25445434948527));
#22926=CARTESIAN_POINT('',(49.160334755135,3.63165946910083,0.924458462629187));
#22927=CARTESIAN_POINT('Origin',(49.1370633864693,3.63165946910083,1.42391661242798));
#22928=CARTESIAN_POINT('',(49.160334755135,-3.63165946910082,0.924458462629194));
#22929=CARTESIAN_POINT('',(48.6666566035268,-3.63165946910082,1.25445434948527));
#22930=CARTESIAN_POINT('Ctrl Pts',(48.6666566035268,3.63165946910083,1.25445434948526));
#22931=CARTESIAN_POINT('Ctrl Pts',(48.6666566035268,3.74656496246816,1.25445434948526));
#22932=CARTESIAN_POINT('Ctrl Pts',(48.6319493120662,4.01324141425168,1.35079760040805));
#22933=CARTESIAN_POINT('Ctrl Pts',(48.541015353828,4.13165946910083,1.60321929012389));
#22934=CARTESIAN_POINT('Ctrl Pts',(48.4890896340131,4.13165946910083,1.74735881939682));
#22935=CARTESIAN_POINT('Ctrl Pts',(48.7025708074101,3.63165946910083,1.1547608553863));
#22936=CARTESIAN_POINT('Ctrl Pts',(48.7025708074101,3.77206824523273,1.1547608553863));
#22937=CARTESIAN_POINT('Ctrl Pts',(48.6621924573285,4.09794567280866,1.26724630381089));
#22938=CARTESIAN_POINT('Ctrl Pts',(48.553613260593,4.25512201950971,1.56895747948715));
#22939=CARTESIAN_POINT('Ctrl Pts',(48.4890896340131,4.2625591630004,1.74735881939682));
#22940=CARTESIAN_POINT('Ctrl Pts',(48.8399066101513,3.63165946910083,0.97936619857827));
#22941=CARTESIAN_POINT('Ctrl Pts',(48.8399066101513,3.82288837992692,0.97936619857827));
#22942=CARTESIAN_POINT('Ctrl Pts',(48.7937718458663,4.26716280005947,1.12633645189498));
#22943=CARTESIAN_POINT('Ctrl Pts',(48.6677634135149,4.50159141936477,1.53315977006196));
#22944=CARTESIAN_POINT('Ctrl Pts',(48.5910979765086,4.52323379775167,1.78410693865264));
#22945=CARTESIAN_POINT('Ctrl Pts',(49.0544843934583,3.63165946910083,0.919526552336082));
#22946=CARTESIAN_POINT('Ctrl Pts',(49.0544843934583,3.85405546772779,0.919526552336082));
#22947=CARTESIAN_POINT('Ctrl Pts',(49.0121746951936,4.37009596294779,1.09945552465902));
#22948=CARTESIAN_POINT('Ctrl Pts',(48.9008757179322,4.61982938830091,1.58461354168167));
#22949=CARTESIAN_POINT('Ctrl Pts',(48.8363442091647,4.63165946910082,1.87245596564607));
#22950=CARTESIAN_POINT('Ctrl Pts',(49.160334755135,3.63165946910083,0.924458462629198));
#22951=CARTESIAN_POINT('Ctrl Pts',(49.160334755135,3.86147045583549,0.924458462629198));
#22952=CARTESIAN_POINT('Ctrl Pts',(49.1200596047313,4.39482335940253,1.11853852679163));
#22953=CARTESIAN_POINT('Ctrl Pts',(49.0170191871873,4.63165946910082,1.6267649545568));
#22954=CARTESIAN_POINT('Ctrl Pts',(48.9594964169557,4.63165946910082,1.91682108233953));
#22955=CARTESIAN_POINT('',(48.4890896340131,4.13165946910083,1.74735881939682));
#22956=CARTESIAN_POINT('',(48.9594964169557,4.63165946910083,1.91682108233953));
#22957=CARTESIAN_POINT('Origin',(48.9594964169557,4.13165946910083,1.91682108233953));
#22958=CARTESIAN_POINT('Ctrl Pts',(48.9594964169557,4.63165946910082,1.91682108233953));
#22959=CARTESIAN_POINT('Ctrl Pts',(49.0170191871873,4.63165946910082,1.6267649545568));
#22960=CARTESIAN_POINT('Ctrl Pts',(49.1200596047313,4.39482335940253,1.11853852679163));
#22961=CARTESIAN_POINT('Ctrl Pts',(49.160334755135,3.86147045583549,0.924458462629198));
#22962=CARTESIAN_POINT('Ctrl Pts',(49.160334755135,3.63165946910083,0.924458462629198));
#22963=CARTESIAN_POINT('Ctrl Pts',(48.6666566035268,3.63165946910083,1.25445434948526));
#22964=CARTESIAN_POINT('Ctrl Pts',(48.6666566035268,3.74656496246816,1.25445434948526));
#22965=CARTESIAN_POINT('Ctrl Pts',(48.6319493120662,4.01324141425168,1.35079760040805));
#22966=CARTESIAN_POINT('Ctrl Pts',(48.541015353828,4.13165946910083,1.60321929012389));
#22967=CARTESIAN_POINT('Ctrl Pts',(48.4890896340131,4.13165946910083,1.74735881939682));
#22968=CARTESIAN_POINT('Origin',(47.6576678782476,4.13165946910082,5.53053993751283));
#22969=CARTESIAN_POINT('',(47.187261095305,4.13165946910082,5.36107767457011));
#22970=CARTESIAN_POINT('',(47.6576678782476,4.63165946910082,5.53053993751283));
#22971=CARTESIAN_POINT('Origin',(46.9750537087877,-3.63165946910082,7.42539446070032));
#22972=CARTESIAN_POINT('',(46.4793852260815,-3.63165946910082,7.49106603180771));
#22973=CARTESIAN_POINT('',(46.9852421795911,-3.63165946910082,7.92529064498532));
#22974=CARTESIAN_POINT('Origin',(57.5530637513316,4.63165946910082,6.17670144644389));
#22975=CARTESIAN_POINT('',(67.849510736113,4.63165946910082,10.0458771867885));
#22976=CARTESIAN_POINT('Origin',(48.2463073637984,4.63165946910082,69.7993133400951));
#22977=CARTESIAN_POINT('',(67.8495107361129,4.63165946910082,9.29710969756502));
#22978=CARTESIAN_POINT('',(67.8495107361129,4.63165946910082,7.38584475819711));
#22979=CARTESIAN_POINT('',(59.746010728986,4.63165946910082,5.83920248277193));
#22980=CARTESIAN_POINT('Ctrl Pts',(59.746010728986,4.63165946910082,5.83920248277193));
#22981=CARTESIAN_POINT('Ctrl Pts',(59.7553520150816,4.63165946910082,5.84546856158671));
#22982=CARTESIAN_POINT('Ctrl Pts',(59.7646938885029,4.63165946910082,5.85173542775135));
#22983=CARTESIAN_POINT('Ctrl Pts',(60.2628303227855,4.63165946910084,6.1858477117844));
#22984=CARTESIAN_POINT('Ctrl Pts',(61.2531647920567,4.63165946910082,6.82066652204582));
#22985=CARTESIAN_POINT('Ctrl Pts',(62.8100479900584,4.63165946910083,7.66426081171851));
#22986=CARTESIAN_POINT('Ctrl Pts',(64.4774359515706,4.63165946910083,8.25725916914412));
#22987=CARTESIAN_POINT('Ctrl Pts',(66.1709303349025,4.63165946910083,8.74915286435064));
#22988=CARTESIAN_POINT('Ctrl Pts',(67.2933262825326,4.63165946910082,9.10437306478713));
#22989=CARTESIAN_POINT('Ctrl Pts',(67.8495107361129,4.63165946910082,9.29710969756502));
#22990=CARTESIAN_POINT('Origin',(48.2394105756736,4.63165946910082,20.6896511931003));
#22991=CARTESIAN_POINT('Origin',(48.2463073637984,3.63165946910083,69.7993133400951));
#22992=CARTESIAN_POINT('',(67.5377890263469,3.63165946910083,10.9960506318292));
#22993=CARTESIAN_POINT('Origin',(48.2463073637984,3.63165946910083,69.7993133400951));
#22994=CARTESIAN_POINT('Origin',(67.849510736113,3.63165946910083,10.0458771867885));
#22995=CARTESIAN_POINT('Origin',(48.2463073637984,-3.63165946910082,69.7993133400951));
#22996=CARTESIAN_POINT('',(67.5377890263469,-3.63165946910083,10.9960506318292));
#22997=CARTESIAN_POINT('Origin',(48.2463073637984,-3.63165946910083,69.7993133400951));
#22998=CARTESIAN_POINT('',(67.5377890263469,-3.63165946910082,10.9960506318292));
#22999=CARTESIAN_POINT('Origin',(48.2463073637984,-3.63165946910083,69.7993133400951));
#23000=CARTESIAN_POINT('',(67.849510736113,-4.63165946910082,10.0458771867885));
#23001=CARTESIAN_POINT('Origin',(48.2463073637984,-4.63165946910082,69.7993133400951));
#23002=CARTESIAN_POINT('Origin',(67.849510736113,-3.63165946910083,10.0458771867885));
#23003=CARTESIAN_POINT('Origin',(46.2566167665501,-3.63165946910082,7.94443397556152));
#23004=CARTESIAN_POINT('',(48.6333391993365,-3.63165946910082,1.34693944114521));
#23005=CARTESIAN_POINT('',(46.2566167665501,-3.63165946910082,7.94443397556152));
#23006=CARTESIAN_POINT('',(48.6333391993365,3.63165946910082,1.3469394411452));
#23007=CARTESIAN_POINT('',(48.6333391993365,-3.63165946910082,1.34693944114521));
#23008=CARTESIAN_POINT('',(46.2566167665501,3.63165946910082,7.94443397556152));
#23009=CARTESIAN_POINT('Ctrl Pts',(60.3030816362698,-3.63165946910082,5.00873755018416));
#23010=CARTESIAN_POINT('Ctrl Pts',(60.3124229223654,-3.63165946910082,5.01500362899892));
#23011=CARTESIAN_POINT('Ctrl Pts',(60.321764208461,-3.63165946910082,5.02126970781368));
#23012=CARTESIAN_POINT('Ctrl Pts',(61.0123101391572,-3.63165946910083,5.48448378590278));
#23013=CARTESIAN_POINT('Ctrl Pts',(62.0505895544972,-3.63165946910083,6.1424866608486));
#23014=CARTESIAN_POINT('Ctrl Pts',(63.4401214267519,-3.63165946910083,6.82140499056667));
#23015=CARTESIAN_POINT('Ctrl Pts',(64.5424665843927,-3.63165946910083,7.2182002185439));
#23016=CARTESIAN_POINT('Ctrl Pts',(65.7313524768425,-3.63165946910082,7.5802308563465));
#23017=CARTESIAN_POINT('Ctrl Pts',(66.9461333967787,-3.63165946910083,7.94539057682941));
#23018=CARTESIAN_POINT('Ctrl Pts',(67.7662134721537,-3.63165946910083,8.20990343773874));
#23019=CARTESIAN_POINT('Ctrl Pts',(68.1769417551788,-3.63165946910083,8.35223461177142));
#23020=CARTESIAN_POINT('Ctrl Pts',(60.3030816362698,-3.93085876944271,5.00873755018416));
#23021=CARTESIAN_POINT('Ctrl Pts',(60.3124229223654,-3.93085876944271,5.01500362899892));
#23022=CARTESIAN_POINT('Ctrl Pts',(60.321764208461,-3.93085876944271,5.02126970781368));
#23023=CARTESIAN_POINT('Ctrl Pts',(61.0123101391572,-3.93085876944271,5.48448378590278));
#23024=CARTESIAN_POINT('Ctrl Pts',(62.0505895544972,-3.93085876944271,6.1424866608486));
#23025=CARTESIAN_POINT('Ctrl Pts',(63.4401214267519,-3.93085876944271,6.82140499056667));
#23026=CARTESIAN_POINT('Ctrl Pts',(64.5424665843927,-3.93085876944271,7.2182002185439));
#23027=CARTESIAN_POINT('Ctrl Pts',(65.7313524768425,-3.93085876944271,7.5802308563465));
#23028=CARTESIAN_POINT('Ctrl Pts',(66.9461333967787,-3.93085876944271,7.94539057682941));
#23029=CARTESIAN_POINT('Ctrl Pts',(67.7662134721537,-3.93085876944271,8.20990343773874));
#23030=CARTESIAN_POINT('Ctrl Pts',(68.1769417551788,-3.93085876944271,8.35223461177142));
#23031=CARTESIAN_POINT('Ctrl Pts',(60.1631225847142,-4.4487252310069,5.21738438992301));
#23032=CARTESIAN_POINT('Ctrl Pts',(60.1724638708098,-4.4487252310069,5.22365046873777));
#23033=CARTESIAN_POINT('Ctrl Pts',(60.1818051569054,-4.4487252310069,5.22991654755253));
#23034=CARTESIAN_POINT('Ctrl Pts',(60.8753903965548,-4.4487252310069,5.69574246490634));
#23035=CARTESIAN_POINT('Ctrl Pts',(61.9223125625907,-4.4487252310069,6.35927401084995));
#23036=CARTESIAN_POINT('Ctrl Pts',(63.3416742095466,-4.4487252310069,7.05326112586659));
#23037=CARTESIAN_POINT('Ctrl Pts',(64.4659491723573,-4.4487252310069,7.45759442605238));
#23038=CARTESIAN_POINT('Ctrl Pts',(65.659435332871,-4.4487252310069,7.82096212027916));
#23039=CARTESIAN_POINT('Ctrl Pts',(66.8721227951014,-4.4487252310069,8.18550871975537));
#23040=CARTESIAN_POINT('Ctrl Pts',(67.6874485389554,-4.4487252310069,8.44852840504606));
#23041=CARTESIAN_POINT('Ctrl Pts',(68.0946776586685,-4.4487252310069,8.58962597275722));
#23042=CARTESIAN_POINT('Ctrl Pts',(59.8710171482611,-4.63165946910083,5.65284658768043));
#23043=CARTESIAN_POINT('Ctrl Pts',(59.8803584343568,-4.63165946910083,5.65911266649519));
#23044=CARTESIAN_POINT('Ctrl Pts',(59.8896997204524,-4.63165946910083,5.66537874530994));
#23045=CARTESIAN_POINT('Ctrl Pts',(60.5926792328869,-4.63165946910082,6.13732137267113));
#23046=CARTESIAN_POINT('Ctrl Pts',(61.6535679847968,-4.63165946910083,6.8114233514931));
#23047=CARTESIAN_POINT('Ctrl Pts',(63.1376324390272,-4.63165946910083,7.53756089343684));
#23048=CARTESIAN_POINT('Ctrl Pts',(64.3069826525201,-4.63165946910083,7.95751277860056));
#23049=CARTESIAN_POINT('Ctrl Pts',(65.509415627788,-4.63165946910082,8.32333666532113));
#23050=CARTESIAN_POINT('Ctrl Pts',(66.7179599089468,-4.63165946910083,8.68677615470624));
#23051=CARTESIAN_POINT('Ctrl Pts',(67.5227731148609,-4.63165946910083,8.94640720339014));
#23052=CARTESIAN_POINT('Ctrl Pts',(67.9229860849654,-4.63165946910083,9.08508022412708));
#23053=CARTESIAN_POINT('Ctrl Pts',(59.7460107289861,-4.63165946910083,5.83920248277199));
#23054=CARTESIAN_POINT('Ctrl Pts',(59.7553520150817,-4.63165946910083,5.84546856158675));
#23055=CARTESIAN_POINT('Ctrl Pts',(59.7646933011773,-4.63165946910083,5.8517346404015));
#23056=CARTESIAN_POINT('Ctrl Pts',(60.4723758535947,-4.63165946910082,6.32644386179577));
#23057=CARTESIAN_POINT('Ctrl Pts',(61.5383304632888,-4.63165946910083,7.00485275615749));
#23058=CARTESIAN_POINT('Ctrl Pts',(63.0506317795768,-4.63165946910083,7.74490586716288));
#23059=CARTESIAN_POINT('Ctrl Pts',(64.2391166337755,-4.63165946910083,8.17151621821202));
#23060=CARTESIAN_POINT('Ctrl Pts',(65.4452319728652,-4.63165946910082,8.53831640988129));
#23061=CARTESIAN_POINT('Ctrl Pts',(66.6520537625864,-4.63165946910083,8.90132071934848));
#23062=CARTESIAN_POINT('Ctrl Pts',(67.4522361264021,-4.63165946910083,9.15944067414874));
#23063=CARTESIAN_POINT('Ctrl Pts',(67.8495107361018,-4.63165946910083,9.29710969756116));
#23064=CARTESIAN_POINT('',(60.331105491743,-3.63165946910083,5.02753578421065));
#23065=CARTESIAN_POINT('',(68.1769417551846,-3.63165946910083,8.35223461177341));
#23066=CARTESIAN_POINT('Ctrl Pts',(60.3311054949517,-3.63165946910082,5.0275357859514));
#23067=CARTESIAN_POINT('Ctrl Pts',(61.0124633196254,-3.63165946910083,5.48458086221223));
#23068=CARTESIAN_POINT('Ctrl Pts',(62.0506664301593,-3.63165946910083,6.14252422191301));
#23069=CARTESIAN_POINT('Ctrl Pts',(63.4401214267519,-3.63165946910083,6.82140499056667));
#23070=CARTESIAN_POINT('Ctrl Pts',(64.5424665843927,-3.63165946910083,7.2182002185439));
#23071=CARTESIAN_POINT('Ctrl Pts',(65.7313524768425,-3.63165946910082,7.5802308563465));
#23072=CARTESIAN_POINT('Ctrl Pts',(66.9461333967787,-3.63165946910083,7.94539057682941));
#23073=CARTESIAN_POINT('Ctrl Pts',(67.7662134721537,-3.63165946910083,8.20990343773874));
#23074=CARTESIAN_POINT('Ctrl Pts',(68.1769417551788,-3.63165946910083,8.35223461177142));
#23075=CARTESIAN_POINT('',(67.8495107361074,-4.63165946910082,9.29710969756116));
#23076=CARTESIAN_POINT('Origin',(67.8495107361018,-3.63165946910083,9.29710969756116));
#23077=CARTESIAN_POINT('',(59.7460107289861,-4.63165946910082,5.839202482772));
#23078=CARTESIAN_POINT('Ctrl Pts',(67.8495107361018,-4.63165946910083,9.29710969756116));
#23079=CARTESIAN_POINT('Ctrl Pts',(67.4522361264021,-4.63165946910083,9.15944067414874));
#23080=CARTESIAN_POINT('Ctrl Pts',(66.6520537625864,-4.63165946910083,8.90132071934848));
#23081=CARTESIAN_POINT('Ctrl Pts',(65.4452319728652,-4.63165946910082,8.53831640988129));
#23082=CARTESIAN_POINT('Ctrl Pts',(64.2391166337755,-4.63165946910083,8.17151621821202));
#23083=CARTESIAN_POINT('Ctrl Pts',(63.0506317795768,-4.63165946910083,7.74490586716288));
#23084=CARTESIAN_POINT('Ctrl Pts',(61.5383304632888,-4.63165946910083,7.00485275615749));
#23085=CARTESIAN_POINT('Ctrl Pts',(60.4723758535947,-4.63165946910082,6.32644386179577));
#23086=CARTESIAN_POINT('Ctrl Pts',(59.7646933011773,-4.63165946910083,5.8517346404015));
#23087=CARTESIAN_POINT('Ctrl Pts',(59.7553520150817,-4.63165946910083,5.84546856158675));
#23088=CARTESIAN_POINT('Ctrl Pts',(59.7460107289861,-4.63165946910083,5.83920248277199));
#23089=CARTESIAN_POINT('Ctrl Pts',(59.7460107289858,-4.63165946910083,5.83920248277159));
#23090=CARTESIAN_POINT('Ctrl Pts',(59.747983173405,-4.63165946910083,5.83760826569162));
#23091=CARTESIAN_POINT('Ctrl Pts',(59.7499465217352,-4.63165033057513,5.83600301592175));
#23092=CARTESIAN_POINT('Ctrl Pts',(59.8106476612128,-4.63108042779695,5.78580377952516));
#23093=CARTESIAN_POINT('Ctrl Pts',(59.8590970533301,-4.62230091506807,5.72906894083519));
#23094=CARTESIAN_POINT('Ctrl Pts',(59.9430417049605,-4.58749976286397,5.60825635642181));
#23095=CARTESIAN_POINT('Ctrl Pts',(59.9774595309507,-4.56225920236549,5.5461849400014));
#23096=CARTESIAN_POINT('Ctrl Pts',(60.0682261303521,-4.47320022945349,5.38630772232757));
#23097=CARTESIAN_POINT('Ctrl Pts',(60.1201210869269,-4.40574630265719,5.31924893308168));
#23098=CARTESIAN_POINT('Ctrl Pts',(60.2084830922883,-4.28319035536618,5.2327413196381));
#23099=CARTESIAN_POINT('Ctrl Pts',(60.27223114969,-4.1877452714611,5.17557566103711));
#23100=CARTESIAN_POINT('Ctrl Pts',(60.320208223554,-3.97475788580983,5.09249114125403));
#23101=CARTESIAN_POINT('Ctrl Pts',(60.3271981253549,-3.90791218641454,5.07054001100713));
#23102=CARTESIAN_POINT('Ctrl Pts',(60.3327487578869,-3.76969211347434,5.03759836393143));
#23103=CARTESIAN_POINT('Ctrl Pts',(60.3311054852527,-3.69976109960378,5.02753577944549));
#23104=CARTESIAN_POINT('Ctrl Pts',(60.3311054852527,-3.63165946910083,5.02753577944548));
#23105=CARTESIAN_POINT('Origin',(67.8495107361129,-3.63165946910083,9.29710969756502));
#23106=CARTESIAN_POINT('',(68.849510736113,-3.63165946910083,9.29710969756497));
#23107=CARTESIAN_POINT('Origin',(67.8495107361129,-3.63165946910083,9.29710969756502));
#23108=CARTESIAN_POINT('Origin',(67.849510736113,-3.63165946910083,9.29710969756502));
#23109=CARTESIAN_POINT('Origin',(48.2394105756736,-3.63165946910083,20.6896511931003));
#23110=CARTESIAN_POINT('Origin',(48.2394105756736,-3.63165946910083,20.6896511931003));
#23111=CARTESIAN_POINT('Origin',(48.2394105756736,-4.63165946910082,20.6896511931003));
#23112=CARTESIAN_POINT('Origin',(67.8495107361129,-3.63165946910083,7.38584475819711));
#23113=CARTESIAN_POINT('',(68.849510736113,-3.63165946910083,10.0458771867885));
#23114=CARTESIAN_POINT('',(68.8495107361129,-3.63165946910083,7.38584475819707));
#23115=CARTESIAN_POINT('Origin',(67.849510736113,-3.63165946910083,10.0458771867885));
#23116=CARTESIAN_POINT('',(67.8495107361129,-4.63165946910082,7.38584475819711));
#23117=CARTESIAN_POINT('Ctrl Pts',(68.849510736113,3.63165946910083,9.29710969756497));
#23118=CARTESIAN_POINT('Ctrl Pts',(68.849510736113,-5.08432325674117,9.29710969756497));
#23119=CARTESIAN_POINT('Ctrl Pts',(68.8495107361129,3.63165946910083,9.09090754844031));
#23120=CARTESIAN_POINT('Ctrl Pts',(68.8495107361129,-5.08432325674117,9.09090754844031));
#23121=CARTESIAN_POINT('Ctrl Pts',(68.7176416128359,3.63165946910083,8.67916780466697));
#23122=CARTESIAN_POINT('Ctrl Pts',(68.7176416128359,-5.08432325674117,8.67916780466697));
#23123=CARTESIAN_POINT('Ctrl Pts',(68.3717770285345,3.63165946910083,8.41975159159924));
#23124=CARTESIAN_POINT('Ctrl Pts',(68.3717770285345,-5.08432325674117,8.41975159159924));
#23125=CARTESIAN_POINT('Ctrl Pts',(68.1769417551904,3.63165946910083,8.3522346117754));
#23126=CARTESIAN_POINT('Ctrl Pts',(68.1769417551904,-5.08432325674117,8.3522346117754));
#23127=CARTESIAN_POINT('',(68.1769417551904,3.63165946910082,8.3522346117754));
#23128=CARTESIAN_POINT('',(68.1769417551904,-3.63165946910084,8.3522346117754));
#23129=CARTESIAN_POINT('',(68.849510736113,3.63165946910083,9.29710969756497));
#23130=CARTESIAN_POINT('Origin',(67.8495107361129,3.63165946910083,9.29710969756502));
#23131=CARTESIAN_POINT('',(68.849510736113,3.63165946910083,9.29710969756497));
#23132=CARTESIAN_POINT('Ctrl Pts',(60.3311054945567,4.63165946910082,5.02753578662844));
#23133=CARTESIAN_POINT('Ctrl Pts',(60.3311054945567,-6.48432325674116,5.02753578662844));
#23134=CARTESIAN_POINT('Ctrl Pts',(60.446720639058,4.63165946910082,5.10508973371974));
#23135=CARTESIAN_POINT('Ctrl Pts',(60.446720639058,-6.48432325674116,5.10508973371974));
#23136=CARTESIAN_POINT('Ctrl Pts',(60.6751612024229,4.63165946910082,5.256858542967));
#23137=CARTESIAN_POINT('Ctrl Pts',(60.6751612024229,-6.48432325674116,5.256858542967));
#23138=CARTESIAN_POINT('Ctrl Pts',(61.0094526814666,4.63165946910082,5.47449446266438));
#23139=CARTESIAN_POINT('Ctrl Pts',(61.0094526814666,-6.48432325674116,5.47449446266438));
#23140=CARTESIAN_POINT('Ctrl Pts',(61.4383158098093,4.63165946910082,5.74449578072259));
#23141=CARTESIAN_POINT('Ctrl Pts',(61.4383158098093,-6.48432325674116,5.74449578072259));
#23142=CARTESIAN_POINT('Ctrl Pts',(61.9466867115244,4.63165946910082,6.04793325275811));
#23143=CARTESIAN_POINT('Ctrl Pts',(61.9466867115244,-6.48432325674116,6.04793325275811));
#23144=CARTESIAN_POINT('Ctrl Pts',(62.4298628019368,4.63165946910082,6.31757162375642));
#23145=CARTESIAN_POINT('Ctrl Pts',(62.4298628019368,-6.48432325674116,6.31757162375642));
#23146=CARTESIAN_POINT('Ctrl Pts',(62.8939157006416,4.63165946910082,6.55518883032436));
#23147=CARTESIAN_POINT('Ctrl Pts',(62.8939157006416,-6.48432325674116,6.55518883032436));
#23148=CARTESIAN_POINT('Ctrl Pts',(63.3503010803271,4.63165946910082,6.76511373244055));
#23149=CARTESIAN_POINT('Ctrl Pts',(63.3503010803271,-6.48432325674116,6.76511373244055));
#23150=CARTESIAN_POINT('Ctrl Pts',(63.817162452721,4.63165946910082,6.95510921550471));
#23151=CARTESIAN_POINT('Ctrl Pts',(63.817162452721,-6.48432325674116,6.95510921550471));
#23152=CARTESIAN_POINT('Ctrl Pts',(64.3144171869106,4.63165946910082,7.13456216129536));
#23153=CARTESIAN_POINT('Ctrl Pts',(64.3144171869106,-6.48432325674116,7.13456216129536));
#23154=CARTESIAN_POINT('Ctrl Pts',(64.8590020041975,4.63165946910082,7.3128881543301));
#23155=CARTESIAN_POINT('Ctrl Pts',(64.8590020041975,-6.48432325674116,7.3128881543301));
#23156=CARTESIAN_POINT('Ctrl Pts',(65.4606023841754,4.63165946910082,7.4980830923353));
#23157=CARTESIAN_POINT('Ctrl Pts',(65.4606023841754,-6.48432325674116,7.4980830923353));
#23158=CARTESIAN_POINT('Ctrl Pts',(66.1152065663236,4.63165946910082,7.69478569974882));
#23159=CARTESIAN_POINT('Ctrl Pts',(66.1152065663236,-6.48432325674116,7.69478569974882));
#23160=CARTESIAN_POINT('Ctrl Pts',(66.8054984748247,4.63165946910082,7.90406632490002));
#23161=CARTESIAN_POINT('Ctrl Pts',(66.8054984748247,-6.48432325674116,7.90406632490002));
#23162=CARTESIAN_POINT('Ctrl Pts',(67.5081873326985,4.63165946910082,8.12495539290683));
#23163=CARTESIAN_POINT('Ctrl Pts',(67.5081873326985,-6.48432325674116,8.12495539290683));
#23164=CARTESIAN_POINT('Ctrl Pts',(68.060936927539,4.63165946910082,8.30930757589414));
#23165=CARTESIAN_POINT('Ctrl Pts',(68.060936927539,-6.48432325674116,8.30930757589414));
#23166=CARTESIAN_POINT('Ctrl Pts',(68.4616084894291,4.63165946910082,8.45095277650561));
#23167=CARTESIAN_POINT('Ctrl Pts',(68.4616084894291,-6.48432325674116,8.45095277650561));
#23168=CARTESIAN_POINT('Ctrl Pts',(68.7214260781516,4.63165946910082,8.54674866119352));
#23169=CARTESIAN_POINT('Ctrl Pts',(68.7214260781516,-6.48432325674116,8.54674866119352));
#23170=CARTESIAN_POINT('Ctrl Pts',(68.8495107361129,4.63165946910082,8.59498806995077));
#23171=CARTESIAN_POINT('Ctrl Pts',(68.8495107361129,-6.48432325674116,8.59498806995077));
#23172=CARTESIAN_POINT('',(60.3311081584417,3.63165946910082,5.02753777349255));
#23173=CARTESIAN_POINT('',(60.3311054945567,-3.63165946910082,5.02753578662843));
#23174=CARTESIAN_POINT('Ctrl Pts',(68.1769417551904,3.63165946910082,8.35223461177543));
#23175=CARTESIAN_POINT('Ctrl Pts',(68.0448580891249,3.63165946910082,8.30646317591714));
#23176=CARTESIAN_POINT('Ctrl Pts',(67.774992316996,3.63165946910082,8.21465783622081));
#23177=CARTESIAN_POINT('Ctrl Pts',(67.3615861901275,3.63165946910082,8.07887174821204));
#23178=CARTESIAN_POINT('Ctrl Pts',(66.8025201331148,3.63165946910082,7.90316336021611));
#23179=CARTESIAN_POINT('Ctrl Pts',(66.1152065663236,3.63165946910082,7.69478569974882));
#23180=CARTESIAN_POINT('Ctrl Pts',(65.4606023841754,3.63165946910082,7.4980830923353));
#23181=CARTESIAN_POINT('Ctrl Pts',(64.8590020041975,3.63165946910082,7.3128881543301));
#23182=CARTESIAN_POINT('Ctrl Pts',(64.3144171869106,3.63165946910082,7.13456216129536));
#23183=CARTESIAN_POINT('Ctrl Pts',(63.817162452721,3.63165946910082,6.95510921550471));
#23184=CARTESIAN_POINT('Ctrl Pts',(63.3503010803271,3.63165946910082,6.76511373244055));
#23185=CARTESIAN_POINT('Ctrl Pts',(62.8939157006416,3.63165946910082,6.55518883032436));
#23186=CARTESIAN_POINT('Ctrl Pts',(62.4298628019368,3.63165946910082,6.31757162375642));
#23187=CARTESIAN_POINT('Ctrl Pts',(61.9466867115244,3.63165946910082,6.04793325275811));
#23188=CARTESIAN_POINT('Ctrl Pts',(61.438316294613,3.63165946910082,5.74449607009322));
#23189=CARTESIAN_POINT('Ctrl Pts',(61.009453703921,3.63165946910082,5.47449510637563));
#23190=CARTESIAN_POINT('Ctrl Pts',(60.6751627963943,3.63165946910082,5.25685958070033));
#23191=CARTESIAN_POINT('Ctrl Pts',(60.4467228175623,3.63165946910082,5.10509118105016));
#23192=CARTESIAN_POINT('Ctrl Pts',(60.331108250942,3.63165946910082,5.02753763559501));
#23193=CARTESIAN_POINT('Origin',(67.849510736113,-3.63165946910083,10.0458771867885));
#23194=CARTESIAN_POINT('Origin',(67.849510736113,-3.63165946910083,10.0458771867885));
#23195=CARTESIAN_POINT('Origin',(57.5530637513316,-4.63165946910082,6.17670144644389));
#23196=CARTESIAN_POINT('Origin',(48.2394105756736,3.63165946910083,20.6896511931003));
#23197=CARTESIAN_POINT('Ctrl Pts',(59.7460107289856,4.63165946910082,5.83920248277122));
#23198=CARTESIAN_POINT('Ctrl Pts',(59.7484213663643,4.63165946910082,5.83791349517356));
#23199=CARTESIAN_POINT('Ctrl Pts',(59.7508238157325,4.63165013641957,5.83661272220212));
#23200=CARTESIAN_POINT('Ctrl Pts',(59.8344558547524,4.63099371608051,5.79074099515917));
#23201=CARTESIAN_POINT('Ctrl Pts',(59.8918098938637,4.61969837883588,5.74011401798109));
#23202=CARTESIAN_POINT('Ctrl Pts',(59.9847123908258,4.58714974455729,5.6393735456099));
#23203=CARTESIAN_POINT('Ctrl Pts',(60.023677918704,4.56201831623123,5.58129068542543));
#23204=CARTESIAN_POINT('Ctrl Pts',(60.1055318301292,4.47921911226623,5.4311154386434));
#23205=CARTESIAN_POINT('Ctrl Pts',(60.1366831105316,4.41377764901186,5.34222783627159));
#23206=CARTESIAN_POINT('Ctrl Pts',(60.2158981698528,4.22648244644917,5.16679346746808));
#23207=CARTESIAN_POINT('Ctrl Pts',(60.2573225934332,4.12722090972173,5.13360448598749));
#23208=CARTESIAN_POINT('Ctrl Pts',(60.2972984071676,4.0012706276777,5.08700751139042));
#23209=CARTESIAN_POINT('Ctrl Pts',(60.3125822841339,3.93012447294352,5.06701348081299));
#23210=CARTESIAN_POINT('Ctrl Pts',(60.3301404264941,3.77717862934284,5.0360516928879));
#23211=CARTESIAN_POINT('Ctrl Pts',(60.3311107648635,3.70172097050662,5.02753985548907));
#23212=CARTESIAN_POINT('Ctrl Pts',(60.3311107648635,3.63165946910082,5.02753985548906));
#23213=CARTESIAN_POINT('Origin',(48.2394105756736,3.63165946910083,20.6896511931003));
#23214=CARTESIAN_POINT('Ctrl Pts',(59.746010728986,4.63165946910082,5.83920248277193));
#23215=CARTESIAN_POINT('Ctrl Pts',(59.7553520150816,4.63165946910082,5.84546856158671));
#23216=CARTESIAN_POINT('Ctrl Pts',(59.7646938885029,4.63165946910082,5.85173542775135));
#23217=CARTESIAN_POINT('Ctrl Pts',(60.2628303227855,4.63165946910084,6.1858477117844));
#23218=CARTESIAN_POINT('Ctrl Pts',(61.2531647920567,4.63165946910082,6.82066652204582));
#23219=CARTESIAN_POINT('Ctrl Pts',(62.8100479900584,4.63165946910083,7.66426081171851));
#23220=CARTESIAN_POINT('Ctrl Pts',(64.4774359515706,4.63165946910083,8.25725916914412));
#23221=CARTESIAN_POINT('Ctrl Pts',(66.1709303349025,4.63165946910083,8.74915286435064));
#23222=CARTESIAN_POINT('Ctrl Pts',(67.2933262825326,4.63165946910082,9.10437306478713));
#23223=CARTESIAN_POINT('Ctrl Pts',(67.8495107361129,4.63165946910082,9.29710969756502));
#23224=CARTESIAN_POINT('Ctrl Pts',(59.9126859546861,4.63165946910083,5.59072795598318));
#23225=CARTESIAN_POINT('Ctrl Pts',(59.9218878363471,4.63165946910083,5.59691875304915));
#23226=CARTESIAN_POINT('Ctrl Pts',(59.9315252774069,4.63165946910082,5.60334758552559));
#23227=CARTESIAN_POINT('Ctrl Pts',(60.4247295228265,4.63165946910084,5.93438604629096));
#23228=CARTESIAN_POINT('Ctrl Pts',(61.4103568228254,4.63165946910082,6.56549663438234));
#23229=CARTESIAN_POINT('Ctrl Pts',(62.932177315481,4.63165946910083,7.38990007808402));
#23230=CARTESIAN_POINT('Ctrl Pts',(64.5615716916243,4.63165946910083,7.96968276822744));
#23231=CARTESIAN_POINT('Ctrl Pts',(66.2581057498348,4.63165946910083,8.46323709414939));
#23232=CARTESIAN_POINT('Ctrl Pts',(67.3846557023474,4.63165946910082,8.81926326169801));
#23233=CARTESIAN_POINT('Ctrl Pts',(67.9474778679311,4.63165946910082,9.01440373298629));
#23234=CARTESIAN_POINT('Ctrl Pts',(60.2011742942814,4.38041846956978,5.16065801989078));
#23235=CARTESIAN_POINT('Ctrl Pts',(60.2104574730015,4.38041846956978,5.16689271932467));
#23236=CARTESIAN_POINT('Ctrl Pts',(60.2200229569978,4.38041846956978,5.17329320559942));
#23237=CARTESIAN_POINT('Ctrl Pts',(60.7084670242163,4.3804184695698,5.50109683581841));
#23238=CARTESIAN_POINT('Ctrl Pts',(61.6806422694785,4.38041846956978,6.12294125446242));
#23239=CARTESIAN_POINT('Ctrl Pts',(63.1462916844765,4.38041846956979,6.91644720799102));
#23240=CARTESIAN_POINT('Ctrl Pts',(64.7063856583534,4.38041846956978,7.4716056430184));
#23241=CARTESIAN_POINT('Ctrl Pts',(66.4093830193833,4.38041846956978,7.9685837608805));
#23242=CARTESIAN_POINT('Ctrl Pts',(67.5450516434801,4.38041846956978,8.32682701341114));
#23243=CARTESIAN_POINT('Ctrl Pts',(68.1170434111871,4.38041846956978,8.52508461568826));
#23244=CARTESIAN_POINT('Ctrl Pts',(60.3030816362697,3.85605894435724,5.0087375501841));
#23245=CARTESIAN_POINT('Ctrl Pts',(60.3124229223653,3.85605894435724,5.01500362899888));
#23246=CARTESIAN_POINT('Ctrl Pts',(60.3219098237078,3.85605894435724,5.02136597894065));
#23247=CARTESIAN_POINT('Ctrl Pts',(60.8090164554297,3.85605894435727,5.34821691824898));
#23248=CARTESIAN_POINT('Ctrl Pts',(61.7759565243552,3.85605894435724,5.96652864430215));
#23249=CARTESIAN_POINT('Ctrl Pts',(63.2221752516257,3.85605894435725,6.74933144341603));
#23250=CARTESIAN_POINT('Ctrl Pts',(64.7574666625901,3.85605894435724,7.29563202006918));
#23251=CARTESIAN_POINT('Ctrl Pts',(66.462856679228,3.85605894435724,7.79386964203506));
#23252=CARTESIAN_POINT('Ctrl Pts',(67.6019221589542,3.85605894435724,8.15297096812908));
#23253=CARTESIAN_POINT('Ctrl Pts',(68.1769417551904,3.85605894435724,8.3522346117754));
#23254=CARTESIAN_POINT('Ctrl Pts',(60.3030816362697,3.63165946910083,5.0087375501841));
#23255=CARTESIAN_POINT('Ctrl Pts',(60.3124229223653,3.63165946910083,5.01500362899888));
#23256=CARTESIAN_POINT('Ctrl Pts',(60.3219098237078,3.63165946910082,5.02136597894065));
#23257=CARTESIAN_POINT('Ctrl Pts',(60.8090164554297,3.63165946910086,5.34821691824898));
#23258=CARTESIAN_POINT('Ctrl Pts',(61.7759565243552,3.63165946910082,5.96652864430215));
#23259=CARTESIAN_POINT('Ctrl Pts',(63.2221752516257,3.63165946910084,6.74933144341603));
#23260=CARTESIAN_POINT('Ctrl Pts',(64.7574666625901,3.63165946910083,7.29563202006918));
#23261=CARTESIAN_POINT('Ctrl Pts',(66.462856679228,3.63165946910083,7.79386964203506));
#23262=CARTESIAN_POINT('Ctrl Pts',(67.6019221589542,3.63165946910082,8.15297096812908));
#23263=CARTESIAN_POINT('Ctrl Pts',(68.1769417551904,3.63165946910082,8.3522346117754));
#23264=CARTESIAN_POINT('Origin',(67.8495107361129,3.63165946910082,9.29710969756502));
#23265=CARTESIAN_POINT('Origin',(67.8495107361129,3.63165946910083,9.29710969756502));
#23266=CARTESIAN_POINT('Origin',(67.8495107361129,3.63165946910083,9.29710969756502));
#23267=CARTESIAN_POINT('Origin',(67.8495107361129,3.63165946910083,7.38584475819711));
#23268=CARTESIAN_POINT('',(68.849510736113,3.63165946910083,10.0458771867885));
#23269=CARTESIAN_POINT('Origin',(67.849510736113,3.63165946910083,10.0458771867885));
#23270=CARTESIAN_POINT('',(68.8495107361129,3.63165946910083,7.38584475819707));
#23271=CARTESIAN_POINT('Origin',(67.849510736113,3.63165946910083,10.0458771867885));
#23272=CARTESIAN_POINT('Origin',(67.849510736113,3.63165946910083,10.0458771867885));
#23273=CARTESIAN_POINT('Origin',(67.849510736113,-3.63165946910082,10.0458771867885));
#23274=CARTESIAN_POINT('',(68.849510736113,-3.63165946910082,10.0458771867885));
#23275=CARTESIAN_POINT('Origin',(68.8495107361129,-3.63165946910082,8.59498806995077));
#23276=CARTESIAN_POINT('Origin',(57.5530637513316,3.63165946910082,6.17670144644389));
#23277=CARTESIAN_POINT('',(68.403087843053,3.63165946910082,8.90436665637973));
#23278=CARTESIAN_POINT('Ctrl Pts',(68.4030878430529,3.63165946910082,8.90436665637969));
#23279=CARTESIAN_POINT('Ctrl Pts',(68.1524251884716,3.63165946910082,8.81037448856025));
#23280=CARTESIAN_POINT('Ctrl Pts',(67.9114447001595,3.63165946910082,8.72240948548772));
#23281=CARTESIAN_POINT('Ctrl Pts',(67.6801396594394,3.63165946910082,8.64046105199615));
#23282=CARTESIAN_POINT('Ctrl Pts',(67.5033958661816,3.63165946910082,8.57784297440588));
#23283=CARTESIAN_POINT('Ctrl Pts',(67.3323019740517,3.63165946910082,8.5187384505674));
#23284=CARTESIAN_POINT('Ctrl Pts',(67.1668319793641,3.63165946910082,8.46311503412855));
#23285=CARTESIAN_POINT('Ctrl Pts',(67.0167717767144,3.63165946910082,8.41267168239798));
#23286=CARTESIAN_POINT('Ctrl Pts',(66.8713371061142,3.63165946910082,8.36509159944541));
#23287=CARTESIAN_POINT('Ctrl Pts',(66.7304811603576,3.63165946910082,8.32031886206648));
#23288=CARTESIAN_POINT('Ctrl Pts',(66.5991138318065,3.63165946910082,8.27856219450235));
#23289=CARTESIAN_POINT('Ctrl Pts',(66.471729349538,3.63165946910082,8.23924762412635));
#23290=CARTESIAN_POINT('Ctrl Pts',(66.3482609420148,3.63165946910082,8.2022969215945));
#23291=CARTESIAN_POINT('Ctrl Pts',(66.2311942728027,3.63165946910082,8.16726208347499));
#23292=CARTESIAN_POINT('Ctrl Pts',(66.1176483084088,3.63165946910082,8.13435255477346));
#23293=CARTESIAN_POINT('Ctrl Pts',(66.0075362307229,3.63165946910082,8.10346765416841));
#23294=CARTESIAN_POINT('Ctrl Pts',(65.9012263499085,3.63165946910082,8.07364921670638));
#23295=CARTESIAN_POINT('Ctrl Pts',(65.7981174703656,3.63165946910082,8.04571817981046));
#23296=CARTESIAN_POINT('Ctrl Pts',(65.6981000899904,3.63165946910082,8.01954833389659));
#23297=CARTESIAN_POINT('Ctrl Pts',(65.6006424733329,3.63165946910082,7.99404825779491));
#23298=CARTESIAN_POINT('Ctrl Pts',(65.5061202399805,3.63165946910082,7.97022047197159));
#23299=CARTESIAN_POINT('Ctrl Pts',(65.4143999331461,3.63165946910082,7.94791197409409));
#23300=CARTESIAN_POINT('Ctrl Pts',(65.3255799119656,3.63165946910082,7.92630889270057));
#23301=CARTESIAN_POINT('Ctrl Pts',(65.2393874705361,3.63165946910082,7.90613058034837));
#23302=CARTESIAN_POINT('Ctrl Pts',(65.1556698865984,3.63165946910082,7.88720280343498));
#23303=CARTESIAN_POINT('Ctrl Pts',(65.07506789503,3.63165946910082,7.86897943334443));
#23304=CARTESIAN_POINT('Ctrl Pts',(64.9967601069725,3.63165946910082,7.85191541352309));
#23305=CARTESIAN_POINT('Ctrl Pts',(64.9205792020063,3.63165946910082,7.83582042303275));
#23306=CARTESIAN_POINT('Ctrl Pts',(64.846118138096,3.63165946910082,7.820088789022));
#23307=CARTESIAN_POINT('Ctrl Pts',(64.7736891723661,3.63165946910082,7.80528312708477));
#23308=CARTESIAN_POINT('Ctrl Pts',(64.7031036424093,3.63165946910082,7.79118902409658));
#23309=CARTESIAN_POINT('Ctrl Pts',(64.6312305851568,3.63165946910082,7.77683783523942));
#23310=CARTESIAN_POINT('Ctrl Pts',(64.5612688955538,3.63165946910082,7.76322441576092));
#23311=CARTESIAN_POINT('Ctrl Pts',(64.492982491524,3.63165946910082,7.7500807655258));
#23312=CARTESIAN_POINT('Ctrl Pts',(64.4224488831997,3.63165946910082,7.73650457725223));
#23313=CARTESIAN_POINT('Ctrl Pts',(64.3537025897904,3.63165946910082,7.72342940546561));
#23314=CARTESIAN_POINT('Ctrl Pts',(64.2864447162966,3.63165946910082,7.71051780525175));
#23315=CARTESIAN_POINT('Ctrl Pts',(64.2131307134005,3.63165946910082,7.69644360031038));
#23316=CARTESIAN_POINT('Ctrl Pts',(64.1415853319417,3.63165946910082,7.68256356416357));
#23317=CARTESIAN_POINT('Ctrl Pts',(64.071374458361,3.63165946910082,7.66839258437265));
#23318=CARTESIAN_POINT('Ctrl Pts',(63.9812801976944,3.63165946910082,7.65020845017701));
#23319=CARTESIAN_POINT('Ctrl Pts',(63.8933827141527,3.63165946910082,7.63154252215813));
#23320=CARTESIAN_POINT('Ctrl Pts',(63.8066895419125,3.63165946910082,7.61131155332181));
#23321=CARTESIAN_POINT('Ctrl Pts',(63.728322356967,3.63165946910082,7.5930235609061));
#23322=CARTESIAN_POINT('Ctrl Pts',(63.6509358784921,3.63165946910082,7.57345251495131));
#23323=CARTESIAN_POINT('Ctrl Pts',(63.57378242349,3.63165946910082,7.55181695935026));
#23324=CARTESIAN_POINT('Ctrl Pts',(63.5094090616368,3.63165946910082,7.53376522790721));
#23325=CARTESIAN_POINT('Ctrl Pts',(63.4451971003337,3.63165946910082,7.51427577290783));
#23326=CARTESIAN_POINT('Ctrl Pts',(63.3807236660863,3.63165946910082,7.49293131763497));
#23327=CARTESIAN_POINT('Ctrl Pts',(63.3224846953064,3.63165946910082,7.47365083224652));
#23328=CARTESIAN_POINT('Ctrl Pts',(63.2640320091646,3.63165946910082,7.45285644728535));
#23329=CARTESIAN_POINT('Ctrl Pts',(63.2050711081345,3.63165946910082,7.43027832497762));
#23330=CARTESIAN_POINT('Ctrl Pts',(63.1502701886774,3.63165946910082,7.40929320025156));
#23331=CARTESIAN_POINT('Ctrl Pts',(63.0950299666058,3.63165946910082,7.38676687657799));
#23332=CARTESIAN_POINT('Ctrl Pts',(63.0391341137597,3.63165946910082,7.36252141714122));
#23333=CARTESIAN_POINT('Ctrl Pts',(62.9856894260991,3.63165946910082,7.33933917837381));
#23334=CARTESIAN_POINT('Ctrl Pts',(62.9316451194371,3.63165946910082,7.31458499408552));
#23335=CARTESIAN_POINT('Ctrl Pts',(62.8768347758996,3.63165946910082,7.28814419321545));
#23336=CARTESIAN_POINT('Ctrl Pts',(62.821749297725,3.63165946910082,7.26157066593498));
#23337=CARTESIAN_POINT('Ctrl Pts',(62.7658899881053,3.63165946910082,7.23329348079273));
#23338=CARTESIAN_POINT('Ctrl Pts',(62.7091146273812,3.63165946910082,7.20324266246051));
#23339=CARTESIAN_POINT('Ctrl Pts',(62.6513638361753,3.63165946910082,7.17267555530464));
#23340=CARTESIAN_POINT('Ctrl Pts',(62.5926652593515,3.63165946910082,7.14027344884607));
#23341=CARTESIAN_POINT('Ctrl Pts',(62.5328969217323,3.63165946910082,7.10600964833574));
#23342=CARTESIAN_POINT('Ctrl Pts',(62.4718828857829,3.63165946910082,7.07103171789008));
#23343=CARTESIAN_POINT('Ctrl Pts',(62.4097540366417,3.63165946910082,7.03411378207533));
#23344=CARTESIAN_POINT('Ctrl Pts',(62.3464091406167,3.63165946910082,6.99527446217524));
#23345=CARTESIAN_POINT('Ctrl Pts',(62.2811210251423,3.63165946910082,6.95524367577082));
#23346=CARTESIAN_POINT('Ctrl Pts',(62.2145411445452,3.63165946910082,6.91317198799666));
#23347=CARTESIAN_POINT('Ctrl Pts',(62.1465884817725,3.63165946910082,6.86912731598505));
#23348=CARTESIAN_POINT('Ctrl Pts',(62.0761205275452,3.63165946910082,6.82345231511491));
#23349=CARTESIAN_POINT('Ctrl Pts',(62.0041763233329,3.63165946910082,6.7756557855778));
#23350=CARTESIAN_POINT('Ctrl Pts',(61.9306965406046,3.63165946910082,6.72586077918759));
#23351=CARTESIAN_POINT('Ctrl Pts',(61.8540789578711,3.63165946910082,6.67393938148928));
#23352=CARTESIAN_POINT('Ctrl Pts',(61.7757918913736,3.63165946910082,6.61984545880833));
#23353=CARTESIAN_POINT('Ctrl Pts',(61.6958005596679,3.63165946910082,6.56376514048228));
#23354=CARTESIAN_POINT('Ctrl Pts',(61.6117739636066,3.63165946910082,6.50485577924902));
#23355=CARTESIAN_POINT('Ctrl Pts',(61.5258668448555,3.63165946910082,6.44375490099631));
#23356=CARTESIAN_POINT('Ctrl Pts',(61.4380735612011,3.63165946910082,6.38072390991561));
#23357=CARTESIAN_POINT('Ctrl Pts',(61.3405968077594,3.63165946910082,6.31074069342094));
#23358=CARTESIAN_POINT('Ctrl Pts',(61.2407946053347,3.63165946910082,6.23837837095361));
#23359=CARTESIAN_POINT('Ctrl Pts',(61.1387033051201,3.63165946910082,6.16404542577452));
#23360=CARTESIAN_POINT('Ctrl Pts',(61.0257726543044,3.63165946910082,6.08182032080983));
#23361=CARTESIAN_POINT('Ctrl Pts',(60.9100409429449,3.63165946910082,5.99718492622526));
#23362=CARTESIAN_POINT('Ctrl Pts',(60.7916116265055,3.63165946910082,5.910741059164));
#23363=CARTESIAN_POINT('Ctrl Pts',(60.6580479108045,3.63165946910082,5.81325029900941));
#23364=CARTESIAN_POINT('Ctrl Pts',(60.5210532648285,3.63165946910082,5.71346202414252));
#23365=CARTESIAN_POINT('Ctrl Pts',(60.3808417449914,3.63165946910082,5.61226971445713));
#23366=CARTESIAN_POINT('Ctrl Pts',(60.2543711859363,3.63165946910082,5.52099441844102));
#23367=CARTESIAN_POINT('Ctrl Pts',(60.1252852457356,3.63165946910082,5.42857957892073));
#23368=CARTESIAN_POINT('Ctrl Pts',(59.9937718372108,3.63165946910082,5.33566159665948));
#23369=CARTESIAN_POINT('Ctrl Pts',(59.8714966547022,3.63165946910082,5.24927068514123));
#23370=CARTESIAN_POINT('Ctrl Pts',(59.7471238625868,3.63165946910082,5.16244575286178));
#23371=CARTESIAN_POINT('Ctrl Pts',(59.6208147984602,3.63165946910082,5.07565516314998));
#23372=CARTESIAN_POINT('Ctrl Pts',(59.4982169131285,3.63165946910082,4.99141463109531));
#23373=CARTESIAN_POINT('Ctrl Pts',(59.3737951905991,3.63165946910082,4.90720667908688));
#23374=CARTESIAN_POINT('Ctrl Pts',(59.247700268628,3.63165946910082,4.82341149904876));
#23375=CARTESIAN_POINT('Ctrl Pts',(59.1205071392074,3.63165946910082,4.73888651570445));
#23376=CARTESIAN_POINT('Ctrl Pts',(58.9916117176436,3.63165946910082,4.65478168438331));
#23377=CARTESIAN_POINT('Ctrl Pts',(58.8611677026219,3.63165946910082,4.57143304088211));
#23378=CARTESIAN_POINT('Ctrl Pts',(58.7268954605109,3.63165946910082,4.48563830941861));
#23379=CARTESIAN_POINT('Ctrl Pts',(58.5909824288711,3.63165946910082,4.4006446245073));
#23380=CARTESIAN_POINT('Ctrl Pts',(58.4535940638078,3.63165946910082,4.31676247264537));
#23381=CARTESIAN_POINT('Ctrl Pts',(58.3135767950974,3.63165946910082,4.23127524967813));
#23382=CARTESIAN_POINT('Ctrl Pts',(58.172027277087,3.63165946910082,4.14694233221852));
#23383=CARTESIAN_POINT('Ctrl Pts',(58.0291176860168,3.63165946910082,4.06403836576243));
#23384=CARTESIAN_POINT('Ctrl Pts',(57.8844984402709,3.63165946910082,3.9801426033546));
#23385=CARTESIAN_POINT('Ctrl Pts',(57.7384865353406,3.63165946910083,3.8977101052527));
#23386=CARTESIAN_POINT('Ctrl Pts',(57.5912554524475,3.63165946910083,3.81697225280899));
#23387=CARTESIAN_POINT('Ctrl Pts',(57.4411855775284,3.63165946910083,3.73467767764605));
#23388=CARTESIAN_POINT('Ctrl Pts',(57.2898492019476,3.63165946910083,3.65414360653815));
#23389=CARTESIAN_POINT('Ctrl Pts',(57.1374225697492,3.63165946910083,3.575561274548));
#23390=CARTESIAN_POINT('Ctrl Pts',(56.9812329132406,3.63165946910083,3.49503894544995));
#23391=CARTESIAN_POINT('Ctrl Pts',(56.82389865689,3.63165946910083,3.41656573389789));
#23392=CARTESIAN_POINT('Ctrl Pts',(56.6655994249122,3.63165946910083,3.340293868234));
#23393=CARTESIAN_POINT('Ctrl Pts',(56.501946506452,3.63165946910083,3.2614424849623));
#23394=CARTESIAN_POINT('Ctrl Pts',(56.3372624700534,3.63165946910083,3.18494377213621));
#23395=CARTESIAN_POINT('Ctrl Pts',(56.1717322849393,3.63165946910083,3.11091154608564));
#23396=CARTESIAN_POINT('Ctrl Pts',(56.0024276869476,3.63165946910083,3.03519124008049));
#23397=CARTESIAN_POINT('Ctrl Pts',(55.8322381664413,3.63165946910083,2.96205096200203));
#23398=CARTESIAN_POINT('Ctrl Pts',(55.6613439821123,3.63165946910083,2.89155902627219));
#23399=CARTESIAN_POINT('Ctrl Pts',(55.4861649710066,3.63165946910083,2.81929964751945));
#23400=CARTESIAN_POINT('Ctrl Pts',(55.3102457891247,3.63165946910083,2.74982277944709));
#23401=CARTESIAN_POINT('Ctrl Pts',(55.1337581760356,3.63165946910083,2.68315043469479));
#23402=CARTESIAN_POINT('Ctrl Pts',(54.9532225222413,3.63165946910083,2.61494884740395));
#23403=CARTESIAN_POINT('Ctrl Pts',(54.7720923867629,3.63165946910083,2.54968152006114));
#23404=CARTESIAN_POINT('Ctrl Pts',(54.5905239270766,3.63165946910083,2.48732409656624));
#23405=CARTESIAN_POINT('Ctrl Pts',(54.4052967110213,3.63165946910083,2.42371011881756));
#23406=CARTESIAN_POINT('Ctrl Pts',(54.2196137418316,3.63165946910082,2.36312402272515));
#23407=CARTESIAN_POINT('Ctrl Pts',(54.0336065701925,3.63165946910082,2.30549732676221));
#23408=CARTESIAN_POINT('Ctrl Pts',(53.8387224059876,3.63165946910082,2.24512045860351));
#23409=CARTESIAN_POINT('Ctrl Pts',(53.6434823245496,3.63165946910083,2.18799183172259));
#23410=CARTESIAN_POINT('Ctrl Pts',(53.4479954020231,3.63165946910083,2.13399288221745));
#23411=CARTESIAN_POINT('Ctrl Pts',(53.2249151702052,3.63165946910083,2.07237188978564));
#23412=CARTESIAN_POINT('Ctrl Pts',(53.0015135292926,3.63165946910083,2.01482634101555));
#23413=CARTESIAN_POINT('Ctrl Pts',(52.7778983586911,3.63165946910083,1.96113227115105));
#23414=CARTESIAN_POINT('Ctrl Pts',(52.5225551474507,3.63165946910083,1.89981972161835));
#23415=CARTESIAN_POINT('Ctrl Pts',(52.2669323001051,3.63165946910083,1.84352809056697));
#23416=CARTESIAN_POINT('Ctrl Pts',(52.0111327763155,3.63165946910083,1.79187414000036));
#23417=CARTESIAN_POINT('Ctrl Pts',(51.7291129942993,3.63165946910083,1.73492549653435));
#23418=CARTESIAN_POINT('Ctrl Pts',(51.4468750698643,3.63165946910083,1.68361086005454));
#23419=CARTESIAN_POINT('Ctrl Pts',(51.1645293729854,3.63165946910083,1.63739431772361));
#23420=CARTESIAN_POINT('Ctrl Pts',(50.9361416709355,3.63165946910083,1.60001004016484));
#23421=CARTESIAN_POINT('Ctrl Pts',(50.7076817864648,3.63165946910083,1.5659600732803));
#23422=CARTESIAN_POINT('Ctrl Pts',(50.4792240082351,3.63165946910083,1.53497655175055));
#23423=CARTESIAN_POINT('Ctrl Pts',(50.2700379291693,3.63165946910083,1.50660666461129));
#23424=CARTESIAN_POINT('Ctrl Pts',(50.0608529569732,3.63165946910083,1.48080711340197));
#23425=CARTESIAN_POINT('Ctrl Pts',(49.8517551192908,3.63165946910083,1.45739919122166));
#23426=CARTESIAN_POINT('Ctrl Pts',(49.648357764131,3.63165946910083,1.43462942222725));
#23427=CARTESIAN_POINT('Ctrl Pts',(49.4450421707224,3.63165946910083,1.41412203464256));
#23428=CARTESIAN_POINT('Ctrl Pts',(49.2419255557958,3.63165946910083,1.39574767539995));
#23429=CARTESIAN_POINT('Ctrl Pts',(49.0608871158299,3.63165946910083,1.37937055463186));
#23430=CARTESIAN_POINT('Ctrl Pts',(48.8800066915195,3.63165946910083,1.36468794115039));
#23431=CARTESIAN_POINT('Ctrl Pts',(48.6994022361495,3.63165946910082,1.35164010884257));
#23432=CARTESIAN_POINT('Ctrl Pts',(48.6773769868982,3.63165946910082,1.35004888697497));
#23433=CARTESIAN_POINT('Ctrl Pts',(48.6553558896734,3.63165946910082,1.34848202152824));
#23434=CARTESIAN_POINT('Ctrl Pts',(48.6333391993365,3.63165946910082,1.3469394411452));
#23435=CARTESIAN_POINT('',(68.4030878430531,3.63165946910082,10.8150451223525));
#23436=CARTESIAN_POINT('',(68.4030878430529,3.63165946910082,7.54053405141158));
#23437=CARTESIAN_POINT('Origin',(48.2463073637984,3.63165946910082,69.7993133400951));
#23438=CARTESIAN_POINT('Origin',(48.2463073637984,-3.63165946910082,69.7993133400951));
#23439=CARTESIAN_POINT('',(68.4030878430531,-3.63165946910082,10.8150451223525));
#23440=CARTESIAN_POINT('',(68.4030878430531,-3.63165946910082,10.8150451223525));
#23441=CARTESIAN_POINT('Origin',(48.2463073637984,-3.63165946910082,69.7993133400951));
#23442=CARTESIAN_POINT('Origin',(68.403087843053,-3.63165946910082,8.90436665637973));
#23443=CARTESIAN_POINT('',(68.403087843053,-3.63165946910082,8.90436665637973));
#23444=CARTESIAN_POINT('',(68.403087843053,-3.63165946910082,8.90436665637973));
#23445=CARTESIAN_POINT('',(68.4030878430529,-3.63165946910082,7.54053405141158));
#23446=CARTESIAN_POINT('Ctrl Pts',(48.6333391993365,-3.63165946910083,1.3469394411452));
#23447=CARTESIAN_POINT('Ctrl Pts',(48.6333391993365,5.68394053089918,1.3469394411452));
#23448=CARTESIAN_POINT('Ctrl Pts',(48.6559901910909,-3.63165946910083,1.34852646330893));
#23449=CARTESIAN_POINT('Ctrl Pts',(48.6559901910909,5.68394053089918,1.34852646330893));
#23450=CARTESIAN_POINT('Ctrl Pts',(48.8580826500258,-3.63165946910082,1.3628745531293));
#23451=CARTESIAN_POINT('Ctrl Pts',(48.8580826500258,5.68394053089919,1.3628745531293));
#23452=CARTESIAN_POINT('Ctrl Pts',(49.2401770875181,-3.63165946910082,1.3931854505195));
#23453=CARTESIAN_POINT('Ctrl Pts',(49.2401770875181,5.68394053089919,1.3931854505195));
#23454=CARTESIAN_POINT('Ctrl Pts',(49.8030694790913,-3.63165946910082,1.44683819965743));
#23455=CARTESIAN_POINT('Ctrl Pts',(49.8030694790913,5.68394053089919,1.44683819965743));
#23456=CARTESIAN_POINT('Ctrl Pts',(50.5469014142808,-3.63165946910082,1.53623826938649));
#23457=CARTESIAN_POINT('Ctrl Pts',(50.5469014142808,5.68394053089919,1.53623826938649));
#23458=CARTESIAN_POINT('Ctrl Pts',(51.4480843800216,-3.63165946910082,1.67655609650635));
#23459=CARTESIAN_POINT('Ctrl Pts',(51.4480843800216,5.68394053089919,1.67655609650635));
#23460=CARTESIAN_POINT('Ctrl Pts',(52.348266859532,-3.63165946910082,1.85267033982542));
#23461=CARTESIAN_POINT('Ctrl Pts',(52.348266859532,5.68394053089919,1.85267033982542));
#23462=CARTESIAN_POINT('Ctrl Pts',(53.2467046577141,-3.63165946910082,2.06850649471347));
#23463=CARTESIAN_POINT('Ctrl Pts',(53.2467046577141,5.68394053089919,2.06850649471347));
#23464=CARTESIAN_POINT('Ctrl Pts',(54.1422176988182,-3.63165946910082,2.32761261079463));
#23465=CARTESIAN_POINT('Ctrl Pts',(54.1422176988182,5.68394053089919,2.32761261079463));
#23466=CARTESIAN_POINT('Ctrl Pts',(55.0326050724517,-3.63165946910082,2.63265678969324));
#23467=CARTESIAN_POINT('Ctrl Pts',(55.0326050724517,5.68394053089919,2.63265678969324));
#23468=CARTESIAN_POINT('Ctrl Pts',(55.9141550877392,-3.63165946910082,2.98491249335729));
#23469=CARTESIAN_POINT('Ctrl Pts',(55.9141550877392,5.68394053089919,2.98491249335729));
#23470=CARTESIAN_POINT('Ctrl Pts',(56.7819405807955,-3.63165946910082,3.3836558364077));
#23471=CARTESIAN_POINT('Ctrl Pts',(56.7819405807955,5.68394053089919,3.3836558364077));
#23472=CARTESIAN_POINT('Ctrl Pts',(57.6300359536437,-3.63165946910082,3.82554246975634));
#23473=CARTESIAN_POINT('Ctrl Pts',(57.6300359536437,5.68394053089919,3.82554246975634));
#23474=CARTESIAN_POINT('Ctrl Pts',(58.4517774296143,-3.63165946910082,4.30403237376386));
#23475=CARTESIAN_POINT('Ctrl Pts',(58.4517774296143,5.68394053089919,4.30403237376386));
#23476=CARTESIAN_POINT('Ctrl Pts',(59.2399671195477,-3.63165946910082,4.80867544303911));
#23477=CARTESIAN_POINT('Ctrl Pts',(59.2399671195477,5.68394053089919,4.80867544303911));
#23478=CARTESIAN_POINT('Ctrl Pts',(59.9871842641414,-3.63165946910082,5.32469977859742));
#23479=CARTESIAN_POINT('Ctrl Pts',(59.9871842641414,5.68394053089919,5.32469977859742));
#23480=CARTESIAN_POINT('Ctrl Pts',(60.6858451039897,-3.63165946910082,5.83183545124052));
#23481=CARTESIAN_POINT('Ctrl Pts',(60.6858451039897,5.68394053089919,5.83183545124052));
#23482=CARTESIAN_POINT('Ctrl Pts',(61.3291075829706,-3.63165946910082,6.30568784052758));
#23483=CARTESIAN_POINT('Ctrl Pts',(61.3291075829706,5.68394053089919,6.30568784052758));
#23484=CARTESIAN_POINT('Ctrl Pts',(61.9129286688635,-3.63165946910082,6.72264590044013));
#23485=CARTESIAN_POINT('Ctrl Pts',(61.9129286688635,5.68394053089919,6.72264590044013));
#23486=CARTESIAN_POINT('Ctrl Pts',(62.4378966914009,-3.63165946910082,7.06401270956655));
#23487=CARTESIAN_POINT('Ctrl Pts',(62.4378966914009,5.68394053089919,7.06401270956655));
#23488=CARTESIAN_POINT('Ctrl Pts',(62.9110626727188,-3.63165946910082,7.32028203996567));
#23489=CARTESIAN_POINT('Ctrl Pts',(62.9110626727188,5.68394053089919,7.32028203996567));
#23490=CARTESIAN_POINT('Ctrl Pts',(63.3480382061253,-3.63165946910082,7.49580221124892));
#23491=CARTESIAN_POINT('Ctrl Pts',(63.3480382061253,5.68394053089919,7.49580221124892));
#23492=CARTESIAN_POINT('Ctrl Pts',(63.7742575841079,-3.63165946910082,7.61203807956635));
#23493=CARTESIAN_POINT('Ctrl Pts',(63.7742575841079,5.68394053089919,7.61203807956635));
#23494=CARTESIAN_POINT('Ctrl Pts',(64.2192519841205,-3.63165946910082,7.69914552267219));
#23495=CARTESIAN_POINT('Ctrl Pts',(64.2192519841205,5.68394053089919,7.69914552267219));
#23496=CARTESIAN_POINT('Ctrl Pts',(64.712086468945,-3.63165946910082,7.78936630198725));
#23497=CARTESIAN_POINT('Ctrl Pts',(64.712086468945,5.68394053089919,7.78936630198725));
#23498=CARTESIAN_POINT('Ctrl Pts',(65.2754113430736,-3.63165946910082,7.90844857460236));
#23499=CARTESIAN_POINT('Ctrl Pts',(65.2754113430736,5.68394053089919,7.90844857460236));
#23500=CARTESIAN_POINT('Ctrl Pts',(65.9237039528771,-3.63165946910082,8.07283920347654));
#23501=CARTESIAN_POINT('Ctrl Pts',(65.9237039528771,5.68394053089919,8.07283920347654));
#23502=CARTESIAN_POINT('Ctrl Pts',(66.6557369297143,-3.63165946910082,8.28958012503505));
#23503=CARTESIAN_POINT('Ctrl Pts',(66.6557369297143,5.68394053089919,8.28958012503505));
#23504=CARTESIAN_POINT('Ctrl Pts',(67.3150092482541,-3.63165946910082,8.50886642156034));
#23505=CARTESIAN_POINT('Ctrl Pts',(67.3150092482541,5.68394053089919,8.50886642156034));
#23506=CARTESIAN_POINT('Ctrl Pts',(67.8492602326033,-3.63165946910082,8.69890399191604));
#23507=CARTESIAN_POINT('Ctrl Pts',(67.8492602326033,5.68394053089919,8.69890399191604));
#23508=CARTESIAN_POINT('Ctrl Pts',(68.2198703338295,-3.63165946910082,8.8356647155056));
#23509=CARTESIAN_POINT('Ctrl Pts',(68.2198703338295,5.68394053089919,8.8356647155056));
#23510=CARTESIAN_POINT('Ctrl Pts',(68.4030878430529,-3.63165946910082,8.90436665637969));
#23511=CARTESIAN_POINT('Ctrl Pts',(68.4030878430529,5.68394053089919,8.90436665637969));
#23512=CARTESIAN_POINT('Ctrl Pts',(68.4030878430529,-3.63165946910082,8.90436665637969));
#23513=CARTESIAN_POINT('Ctrl Pts',(68.2198703338295,-3.63165946910082,8.8356647155056));
#23514=CARTESIAN_POINT('Ctrl Pts',(67.8492602326033,-3.63165946910082,8.69890399191604));
#23515=CARTESIAN_POINT('Ctrl Pts',(67.3150092482541,-3.63165946910082,8.50886642156034));
#23516=CARTESIAN_POINT('Ctrl Pts',(66.6557369297143,-3.63165946910082,8.28958012503505));
#23517=CARTESIAN_POINT('Ctrl Pts',(65.9237039528771,-3.63165946910082,8.07283920347654));
#23518=CARTESIAN_POINT('Ctrl Pts',(65.2754113430736,-3.63165946910082,7.90844857460236));
#23519=CARTESIAN_POINT('Ctrl Pts',(64.712086468945,-3.63165946910082,7.78936630198725));
#23520=CARTESIAN_POINT('Ctrl Pts',(64.2192519841205,-3.63165946910082,7.69914552267219));
#23521=CARTESIAN_POINT('Ctrl Pts',(63.7742575841079,-3.63165946910082,7.61203807956635));
#23522=CARTESIAN_POINT('Ctrl Pts',(63.3480382061253,-3.63165946910082,7.49580221124892));
#23523=CARTESIAN_POINT('Ctrl Pts',(62.9110626727188,-3.63165946910082,7.32028203996567));
#23524=CARTESIAN_POINT('Ctrl Pts',(62.4378966914009,-3.63165946910082,7.06401270956655));
#23525=CARTESIAN_POINT('Ctrl Pts',(61.9129286688635,-3.63165946910082,6.72264590044013));
#23526=CARTESIAN_POINT('Ctrl Pts',(61.3291075829706,-3.63165946910082,6.30568784052758));
#23527=CARTESIAN_POINT('Ctrl Pts',(60.6858451039897,-3.63165946910082,5.83183545124052));
#23528=CARTESIAN_POINT('Ctrl Pts',(59.9871842641414,-3.63165946910082,5.32469977859742));
#23529=CARTESIAN_POINT('Ctrl Pts',(59.2399671195477,-3.63165946910082,4.80867544303911));
#23530=CARTESIAN_POINT('Ctrl Pts',(58.4517774296143,-3.63165946910082,4.30403237376386));
#23531=CARTESIAN_POINT('Ctrl Pts',(57.6300359536437,-3.63165946910082,3.82554246975634));
#23532=CARTESIAN_POINT('Ctrl Pts',(56.7819405807955,-3.63165946910082,3.3836558364077));
#23533=CARTESIAN_POINT('Ctrl Pts',(55.9141550877392,-3.63165946910082,2.98491249335729));
#23534=CARTESIAN_POINT('Ctrl Pts',(55.0326050724517,-3.63165946910082,2.63265678969324));
#23535=CARTESIAN_POINT('Ctrl Pts',(54.1422176988182,-3.63165946910082,2.32761261079463));
#23536=CARTESIAN_POINT('Ctrl Pts',(53.2467046577141,-3.63165946910082,2.06850649471347));
#23537=CARTESIAN_POINT('Ctrl Pts',(52.348266859532,-3.63165946910082,1.85267033982542));
#23538=CARTESIAN_POINT('Ctrl Pts',(51.4480843800216,-3.63165946910082,1.67655609650635));
#23539=CARTESIAN_POINT('Ctrl Pts',(50.5469014142808,-3.63165946910082,1.53623826938649));
#23540=CARTESIAN_POINT('Ctrl Pts',(49.8030694790913,-3.63165946910082,1.44683819965743));
#23541=CARTESIAN_POINT('Ctrl Pts',(49.2401770875181,-3.63165946910082,1.3931854505195));
#23542=CARTESIAN_POINT('Ctrl Pts',(48.8580826500258,-3.63165946910082,1.3628745531293));
#23543=CARTESIAN_POINT('Ctrl Pts',(48.6559901910909,-3.63165946910083,1.34852646330893));
#23544=CARTESIAN_POINT('Ctrl Pts',(48.6333391993365,-3.63165946910083,1.3469394411452));
#23545=CARTESIAN_POINT('Origin',(57.5530637513316,-3.63165946910082,6.17670144644389));
#23546=CARTESIAN_POINT('Origin',(48.2394105756736,-3.63165946910082,20.6896511931003));
#23565=UNCERTAINTY_MEASURE_WITH_UNIT(LENGTH_MEASURE(0.01),#23578,
'DISTANCE_ACCURACY_VALUE',
'Maximum model space distance between geometric entities at asserted c
onnectivities');
#23566=UNCERTAINTY_MEASURE_WITH_UNIT(LENGTH_MEASURE(0.01),#23578,
'DISTANCE_ACCURACY_VALUE',
'Maximum model space distance between geometric entities at asserted c
onnectivities');
#23576=(
GEOMETRIC_REPRESENTATION_CONTEXT(3)
GLOBAL_UNCERTAINTY_ASSIGNED_CONTEXT((#23565))
GLOBAL_UNIT_ASSIGNED_CONTEXT((#23578,#23580,#23581))
REPRESENTATION_CONTEXT('','3D')
);
#23577=(
GEOMETRIC_REPRESENTATION_CONTEXT(3)
GLOBAL_UNCERTAINTY_ASSIGNED_CONTEXT((#23566))
GLOBAL_UNIT_ASSIGNED_CONTEXT((#23578,#23580,#23581))
REPRESENTATION_CONTEXT('','3D')
);
#23578=(
LENGTH_UNIT()
NAMED_UNIT(*)
SI_UNIT(.MILLI.,.METRE.)
);
#23580=(
NAMED_UNIT(*)
PLANE_ANGLE_UNIT()
SI_UNIT($,.RADIAN.)
);
#23581=(
NAMED_UNIT(*)
SI_UNIT($,.STERADIAN.)
SOLID_ANGLE_UNIT()
);
#23591=SHAPE_DEFINITION_REPRESENTATION(#23601,#23620);
#23601=PRODUCT_DEFINITION_SHAPE('',$,#23631);
#23620=SHAPE_REPRESENTATION('',(#4607),#23576);
#23621=PRODUCT_DEFINITION_CONTEXT('part definition',#23653,'design');
#23631=PRODUCT_DEFINITION('Cover','Cover',#23641,#23621);
#23641=PRODUCT_DEFINITION_FORMATION('',$,#23664);
#23653=APPLICATION_CONTEXT(
'Core Data for Automotive Mechanical Design Process');
#23654=PRODUCT_CONTEXT('part definition',#23653,'mechanical');
#23664=PRODUCT('Cover','Cover',$,(#23654));
#23669=PRESENTATION_STYLE_ASSIGNMENT((#23674));
#23674=SURFACE_STYLE_USAGE(.BOTH.,#23679);
#23679=SURFACE_SIDE_STYLE('',(#23684));
#23684=SURFACE_STYLE_FILL_AREA(#23689);
#23689=FILL_AREA_STYLE('Opaque(144,209,199)',(#23694));
#23694=FILL_AREA_STYLE_COLOUR('Opaque(144,209,199)',#23699);
#23699=COLOUR_RGB('Opaque(144,209,199)', 0.31764706, 0.68627451, 0.89019608);
ENDSEC;
END-ISO-10303-21;
